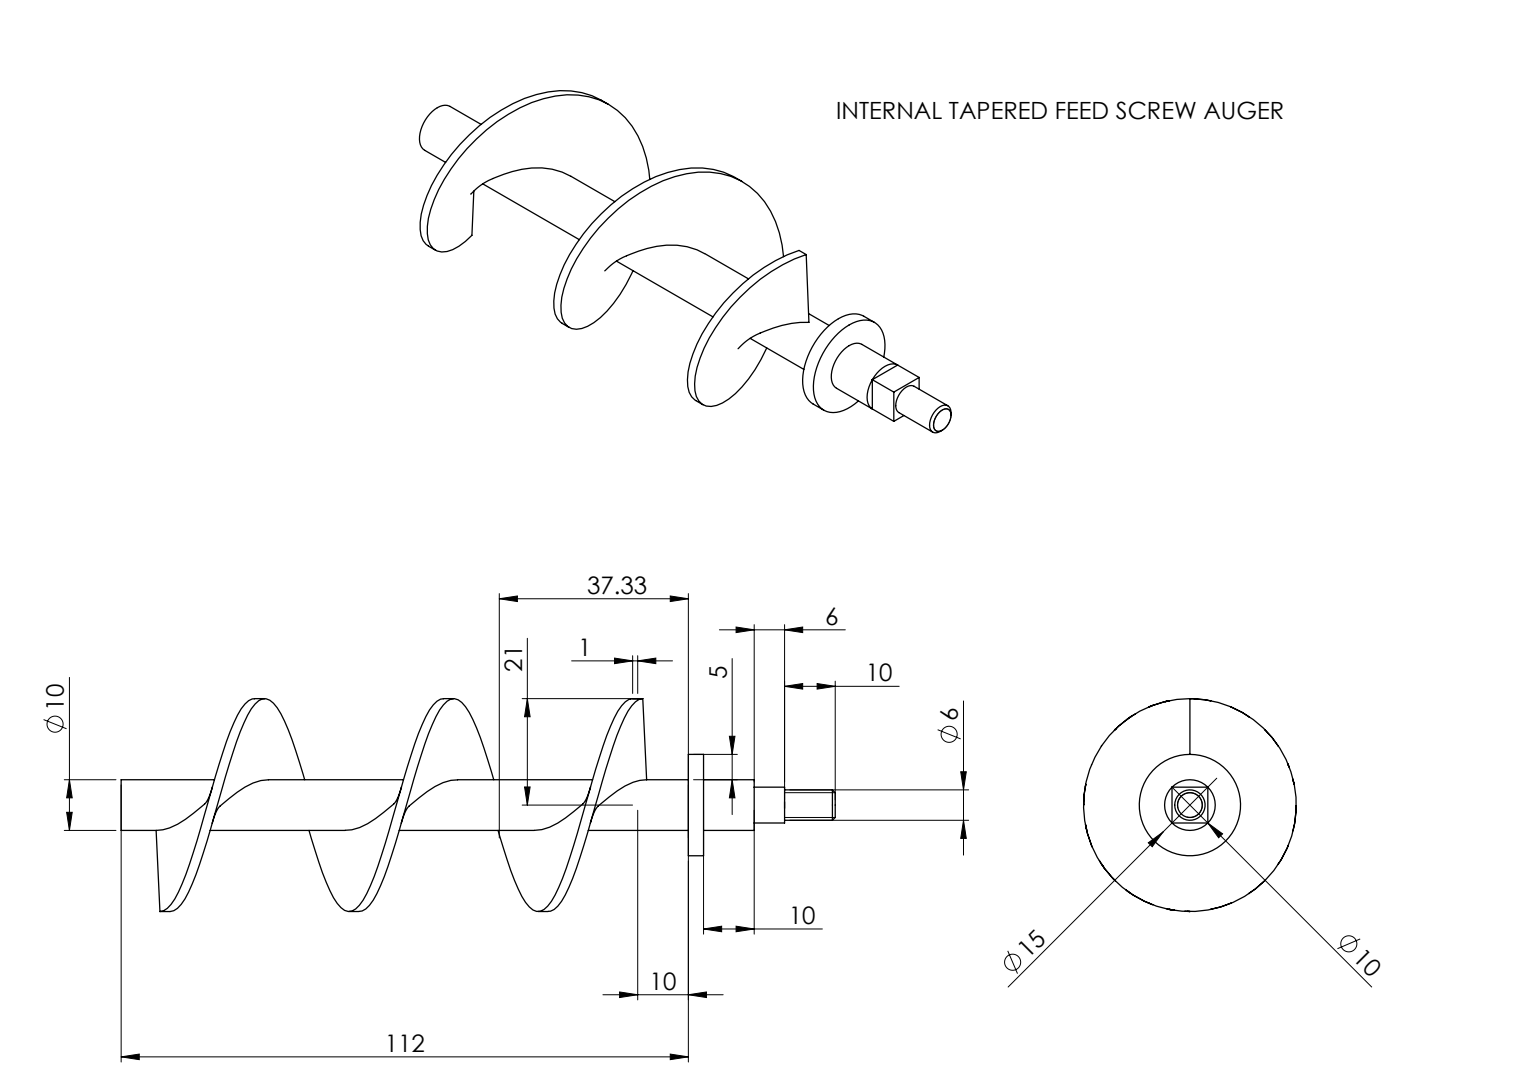
ISO-10303-21;
HEADER;
FILE_DESCRIPTION (('STEP AP214'),
    '1' );
FILE_NAME ('Internal Tapered Feed Screw Auger.step',
    '2026-10-22T10:02:39',
    ( '' ),
    ( '' ),
    'SwSTEP 2.0',
    'SolidWorks 2026',
    '' );
FILE_SCHEMA (( 'AUTOMOTIVE_DESIGN' ));
ENDSEC;

DATA;
#3=CARTESIAN_POINT ( 'NONE',  ( -24.57385867913225042, 55.01967498809302981, -0.01734603766092172178 ) ) ;
#8=CARTESIAN_POINT ( 'NONE',  ( -15.84874342590320673, 58.76832510134365606, 3.302529147201385129 ) ) ;
#12=CARTESIAN_POINT ( 'NONE',  ( 7.477680471578420196, 36.66673471410030061, 10.56605622896702990 ) ) ;
#17=CARTESIAN_POINT ( 'NONE',  ( 3.697305843545918513, 35.98616635274733255, -8.992456113074794644 ) ) ;
#18=EDGE_CURVE ( 'NONE', #2366, #7152, #6007, .T. ) ;
#22=CARTESIAN_POINT ( 'NONE',  ( 18.90732451447525975, 55.01449046109523522, 0.007799356525960917524 ) ) ;
#24=CARTESIAN_POINT ( 'NONE',  ( -46.47759630686348942, 71.80626330759284315, -12.92347896748408509 ) ) ;
#25=CARTESIAN_POINT ( 'NONE',  ( -13.52239577877046095, 75.98118489547775312, -2.745668029642679642 ) ) ;
#32=CARTESIAN_POINT ( 'NONE',  ( -54.99787500575298083, 55.00175321043320764, 0.0009066026748406779724 ) ) ;
#33=CARTESIAN_POINT ( 'NONE',  ( -34.13164850161200548, 51.02358645912743640, -3.048757558511538068 ) ) ;
#38=CARTESIAN_POINT ( 'NONE',  ( -1.477628194636992243, 49.49121550494065502, -20.47411891050684218 ) ) ;
#40=CARTESIAN_POINT ( 'NONE',  ( 10.96071222073927132, 53.39157304099641266, 4.745597011473480009 ) ) ;
#46=CARTESIAN_POINT ( 'NONE',  ( 3.204603673684104592, 51.02314964536983410, -3.048084100943247332 ) ) ;
#47=CARTESIAN_POINT ( 'NONE',  ( -28.33520174651890144, 42.04728119469179148, 5.364820852706460030 ) ) ;
#48=EDGE_CURVE ( 'NONE', #8851, #443, #4129, .T. ) ;
#59=CARTESIAN_POINT ( 'NONE',  ( -47.09272475956910142, 55.02483394329467359, -0.008490977716145282211 ) ) ;
#70=CARTESIAN_POINT ( 'NONE',  ( -62.96917444215183224, 46.00616310598284286, 19.01165851688606523 ) ) ;
#77=CARTESIAN_POINT ( 'NONE',  ( -27.49360061100878738, 37.45598436699922473, 11.71495266747331421 ) ) ;
#80=CARTESIAN_POINT ( 'NONE',  ( -12.37832547621337476, 59.49517489534859749, -2.213937092042313814 ) ) ;
#82=CARTESIAN_POINT ( 'NONE',  ( -3.477628190354089099, 49.49309465598528845, -20.46958112014059950 ) ) ;
#84=CARTESIAN_POINT ( 'NONE',  ( -23.14426256960421924, 52.25445662165124361, 21.02210202263520600 ) ) ;
#85=CARTESIAN_POINT ( 'NONE',  ( -68.81799204399976588, 34.52608862562686909, 5.501299279293338174 ) ) ;
#91=CARTESIAN_POINT ( 'NONE',  ( -44.20488284339200646, 55.00025175640378450, -0.002624240123811788852 ) ) ;
#92=CARTESIAN_POINT ( 'NONE',  ( -56.68145153021548310, 56.29769244905448744, 4.839614506206188160 ) ) ;
#94=CARTESIAN_POINT ( 'NONE',  ( 47.00000000000000000, 55.00000000000000000, 0.000000000000000000 ) ) ;
#95=CARTESIAN_POINT ( 'NONE',  ( -6.249156589778054105, 55.68730665650835476, -7.012895309292545676 ) ) ;
#108=CARTESIAN_POINT ( 'NONE',  ( -34.53957387867419015, 43.82314937793580611, -8.587433708483555250 ) ) ;
#121=CARTESIAN_POINT ( 'NONE',  ( -53.33538954556567546, 54.99810722428492937, -0.002143453996954131253 ) ) ;
#132=CARTESIAN_POINT ( 'NONE',  ( -6.160267096003628318, 59.12214581854949103, -20.69010011304746044 ) ) ;
#136=CARTESIAN_POINT ( 'NONE',  ( -6.214759040711413718, 65.81103152010582846, -18.03762937187994453 ) ) ;
#137=CARTESIAN_POINT ( 'NONE',  ( -46.52239103091250172, 73.32882989972571863, -10.56393531560676102 ) ) ;
#141=CARTESIAN_POINT ( 'NONE',  ( 46.99999999999999289, 58.53553390593273065, 3.535533905932731091 ) ) ;
#142=CARTESIAN_POINT ( 'NONE',  ( 4.636023424558444184, 34.00634798409771520, 1.031279783234476222 ) ) ;
#143=VECTOR ( 'NONE', #3904, 1000.000000000000000 ) ;
#145=CARTESIAN_POINT ( 'NONE',  ( -34.81092923608149192, 36.62878417468885317, -10.58136149031614970 ) ) ;
#146=CARTESIAN_POINT ( 'NONE',  ( -70.34104699118840642, 33.99562393659799397, 0.006612473344882377653 ) ) ;
#149=EDGE_CURVE ( 'NONE', #1776, #658, #10646, .T. ) ;
#151=EDGE_CURVE ( 'NONE', #658, #760, #3805, .T. ) ;
#154=CARTESIAN_POINT ( 'NONE',  ( -35.76380172564871884, 55.01086174631173975, 0.005834152228799136322 ) ) ;
#155=CARTESIAN_POINT ( 'NONE',  ( -44.62221111874860213, 58.76649436596603948, -3.304682393689729381 ) ) ;
#158=CARTESIAN_POINT ( 'NONE',  ( -6.833556764572190190, 56.37289815856257746, -6.894355924324841567 ) ) ;
#161=CARTESIAN_POINT ( 'NONE',  ( 9.477680475861957277, 36.67126955513442255, 10.56417786655960356 ) ) ;
#173=CARTESIAN_POINT ( 'NONE',  ( -30.96365390035560239, 40.99197526476194042, -0.6880654886566857087 ) ) ;
#181=EDGE_LOOP ( 'NONE', ( #6646, #3991, #9037, #3173 ) ) ;
#186=CARTESIAN_POINT ( 'NONE',  ( 6.125158419864718873, 48.06305152834397632, -1.028633690847041704 ) ) ;
#188=DIRECTION ( 'NONE',  ( 0.000000000000000000, 0.000000000000000000, 1.000000000000000000 ) ) ;
#194=CARTESIAN_POINT ( 'NONE',  ( -66.50782127702024127, 36.67013743889115318, 10.55179617378401247 ) ) ;
#197=EDGE_CURVE ( 'NONE', #1911, #3047, #4966, .T. ) ;
#199=CARTESIAN_POINT ( 'NONE',  ( -42.66281101964754896, 63.04450918361814615, -19.42252581123130639 ) ) ;
#200=AXIS2_PLACEMENT_3D ( 'NONE', #7923, #603, #5167 ) ;
#203=CARTESIAN_POINT ( 'NONE',  ( -30.99614452189004155, 33.97742542711323921, 0.0005215828242728561687 ) ) ;
#207=DIRECTION ( 'NONE',  ( -1.000000000000000000, -0.000000000000000000, -0.000000000000000000 ) ) ;
#210=CARTESIAN_POINT ( 'NONE',  ( -56.17294560383920299, 66.73154858138525469, 17.54339796666672058 ) ) ;
#212=CARTESIAN_POINT ( 'NONE',  ( -61.00490302436042356, 55.00059028654953153, 21.02810969917934614 ) ) ;
#215=VECTOR ( 'NONE', #1197, 1000.000000000000000 ) ;
#216=CARTESIAN_POINT ( 'NONE',  ( 53.00000000000000000, 51.46446609406726935, -3.535533905932738197 ) ) ;
#220=CARTESIAN_POINT ( 'NONE',  ( -14.57393009465980604, 54.98364064865898371, -0.001646604999752838971 ) ) ;
#224=CARTESIAN_POINT ( 'NONE',  ( 0.1668379413723253268, 49.14794564670181387, -3.906842406148068214 ) ) ;
#226=CARTESIAN_POINT ( 'NONE',  ( 14.14423903981857755, 49.50929293985068114, 20.43023407247793699 ) ) ;
#228=PLANE ( 'NONE',  #2565 ) ;
#237=CARTESIAN_POINT ( 'NONE',  ( -55.16972311799333539, 62.82217562642412645, 11.69677751401117405 ) ) ;
#246=CARTESIAN_POINT ( 'NONE',  ( -18.95794697780666027, 57.36371471763808927, 6.606639808170175598 ) ) ;
#251=CARTESIAN_POINT ( 'NONE',  ( 52.99999999999999289, 58.53553390593273065, 3.535533905932731091 ) ) ;
#253=CARTESIAN_POINT ( 'NONE',  ( -59.27472368810988002, 61.13901599248961105, 20.20251803659174783 ) ) ;
#256=CARTESIAN_POINT ( 'NONE',  ( -50.82691677660828589, 75.68920158268997511, 4.121780573430135597 ) ) ;
#262=PLANE ( 'NONE',  #3428 ) ;
#266=ADVANCED_FACE ( 'NONE', ( #3949 ), #228, .F. ) ;
#267=CARTESIAN_POINT ( 'NONE',  ( -58.49417186384191325, 59.10997037288393585, 20.69225924102262226 ) ) ;
#268=CARTESIAN_POINT ( 'NONE',  ( 14.87282114002693234, 58.67269055319452065, 13.65170787854068024 ) ) ;
#274=ORIENTED_EDGE ( 'NONE', *, *, #7349, .T. ) ;
#276=CARTESIAN_POINT ( 'NONE',  ( -68.24753854205350478, 55.02494518472502705, -0.0008082322394851507684 ) ) ;
#280=CARTESIAN_POINT ( 'NONE',  ( -69.87738456456679614, 41.01771127808763140, 1.829669757797043994 ) ) ;
#283=CARTESIAN_POINT ( 'NONE',  ( 36.99999999999999289, 59.99999999999998579, 0.000000000000000000 ) ) ;
#284=CARTESIAN_POINT ( 'NONE',  ( 53.00000000000000000, 51.46446609406726935, -3.535533905932738197 ) ) ;
#290=ORIENTED_EDGE ( 'NONE', *, *, #8254, .T. ) ;
#291=EDGE_CURVE ( 'NONE', #2366, #8948, #1373, .T. ) ;
#295=CARTESIAN_POINT ( 'NONE',  ( -53.99820501230367142, 64.90985867132549458, 9.909159326440711624 ) ) ;
#308=CARTESIAN_POINT ( 'NONE',  ( -24.89001229408545512, 50.71618230245203307, 5.579812370254800591 ) ) ;
#310=VECTOR ( 'NONE', #7758, 1000.000000000000227 ) ;
#316=CARTESIAN_POINT ( 'NONE',  ( -63.32723919479404628, 46.95276866351182576, 19.42062151208882170 ) ) ;
#319=CARTESIAN_POINT ( 'NONE',  ( -56.05785376386896246, 64.93131079446247611, 18.59685268580366468 ) ) ;
#321=CARTESIAN_POINT ( 'NONE',  ( -68.34104732181945963, 33.99448141944315438, 0.006743540747239065887 ) ) ;
#324=DIRECTION ( 'NONE',  ( 9.813077866773612233E-16, -1.000000000000000000, 0.000000000000000000 ) ) ;
#325=CARTESIAN_POINT ( 'NONE',  ( 15.18896243380506306, 60.50666922109576262, 20.46968130491651650 ) ) ;
#327=CARTESIAN_POINT ( 'NONE',  ( -61.99390593487224521, 46.95297697149054272, 19.42004845484624909 ) ) ;
#329=CARTESIAN_POINT ( 'NONE',  ( -61.59556246352555320, 52.94114603458827872, 20.93095456750423722 ) ) ;
#336=CARTESIAN_POINT ( 'NONE',  ( -70.57370072173033293, 55.01541170666005343, -0.006042036165150080004 ) ) ;
#339=DIRECTION ( 'NONE',  ( 0.000000000000000000, 0.000000000000000000, 1.000000000000000000 ) ) ;
#340=CARTESIAN_POINT ( 'NONE',  ( 2.791825101730443404, 48.06463389261614338, -1.028630067443766283 ) ) ;
#342=CARTESIAN_POINT ( 'NONE',  ( -28.67054321954914542, 35.57240153874681710, 8.046710727719679213 ) ) ;
#349=EDGE_CURVE ( 'NONE', #1114, #2366, #8625, .T. ) ;
#353=CARTESIAN_POINT ( 'NONE',  ( -58.37019661190561948, 55.68797971655733647, 13.99244826128962593 ) ) ;
#365=EDGE_CURVE ( 'NONE', #1817, #1911, #2263, .T. ) ;
#366=CARTESIAN_POINT ( 'NONE',  ( 5.249530852090826372, 48.30269735457433455, -2.031231156380094660 ) ) ;
#374=ADVANCED_FACE ( 'NONE', ( #6893 ), #4791, .T. ) ;
#376=CARTESIAN_POINT ( 'NONE',  ( -59.82750509709391196, 59.10995506582904824, 20.69284243654335498 ) ) ;
#380=CARTESIAN_POINT ( 'NONE',  ( -59.59556320886013481, 52.94111634316250559, 20.93276532467568174 ) ) ;
#387=CARTESIAN_POINT ( 'NONE',  ( -9.070746587277097817, 68.33487957594263662, -16.24597445391072270 ) ) ;
#389=CARTESIAN_POINT ( 'NONE',  ( 18.18897147127288605, 67.92208482572254979, 16.80535131051722075 ) ) ;
#390=CARTESIAN_POINT ( 'NONE',  ( -3.793771210778672298, 51.32715215846550905, -13.65164055122976983 ) ) ;
#391=DIRECTION ( 'NONE',  ( 6.033820786006286457E-17, -1.000000000000000000, 0.000000000000000000 ) ) ;
#403=CARTESIAN_POINT ( 'NONE',  ( -32.20817489827727087, 48.19891751814265035, 1.703719440855944844 ) ) ;
#405=CARTESIAN_POINT ( 'NONE',  ( -27.49360061100878738, 37.45598436699922473, 11.71495266747331421 ) ) ;
#414=ORIENTED_EDGE ( 'NONE', *, *, #3400, .F. ) ;
#415=CARTESIAN_POINT ( 'NONE',  ( -23.18906244097991021, 49.50939288222085821, 20.43027456479002879 ) ) ;
#428=CARTESIAN_POINT ( 'NONE',  ( -8.750920173525754464, 61.18660372065389907, -3.306409054201195907 ) ) ;
#434=ORIENTED_EDGE ( 'NONE', *, *, #8927, .T. ) ;
#435=CARTESIAN_POINT ( 'NONE',  ( -42.92935705524211443, 57.05913440163546113, -20.93112575922673102 ) ) ;
#443=VERTEX_POINT ( 'NONE', #7009 ) ;
#446=CARTESIAN_POINT ( 'NONE',  ( -32.99614454614441428, 33.97685596767119165, 0.0005149883856687357403 ) ) ;
#449=CARTESIAN_POINT ( 'NONE',  ( -60.26222962708032327, 52.94112624030389469, 20.93216173895077503 ) ) ;
#450=CARTESIAN_POINT ( 'NONE',  ( -25.53957388397973105, 51.34093700237838931, 13.61837799178155350 ) ) ;
#457=CARTESIAN_POINT ( 'NONE',  ( -64.61922394917361601, 54.99794615529658159, 0.004759334053694205813 ) ) ;
#458=VECTOR ( 'NONE', #2991, 1000.000000000000000 ) ;
#461=CARTESIAN_POINT ( 'NONE',  ( -22.00013559226026771, 57.68156399829890546, 6.473040822733857169 ) ) ;
#462=ORIENTED_EDGE ( 'NONE', *, *, #11425, .T. ) ;
#463=CARTESIAN_POINT ( 'NONE',  ( -30.40408068685511367, 34.08504365610654219, 2.058398070974400529 ) ) ;
#473=CARTESIAN_POINT ( 'NONE',  ( -7.070747353360942178, 68.33360022464046324, -16.24461469319379603 ) ) ;
#482=DIRECTION ( 'NONE',  ( -9.813077866773612233E-16, 1.000000000000000000, 0.000000000000000000 ) ) ;
#486=CARTESIAN_POINT ( 'NONE',  ( -60.95809730739352261, 51.99959260526208737, 6.342595581606403243 ) ) ;
#496=LINE ( 'NONE', #7937, #10551 ) ;
#497=CARTESIAN_POINT ( 'NONE',  ( 10.42614132098574586, 55.02481535990867911, -0.008496357143309388182 ) ) ;
#501=CARTESIAN_POINT ( 'NONE',  ( -41.16026710375170694, 50.89060761561553647, -20.69263693287480521 ) ) ;
#503=CARTESIAN_POINT ( 'NONE',  ( -68.19377681732581209, 34.02207046653818168, 2.749122354329981643 ) ) ;
#504=CARTESIAN_POINT ( 'NONE',  ( -41.49691193415848289, 52.26032216745779380, -13.79378832249819986 ) ) ;
#507=CARTESIAN_POINT ( 'NONE',  ( -27.14812531749841895, 52.78402274155275364, 4.494092492992627363 ) ) ;
#511=CARTESIAN_POINT ( 'NONE',  ( -69.75702627179666138, 54.98186149566993208, 0.007223337549123830421 ) ) ;
#514=CIRCLE ( 'NONE', #703, 2.999999999999995559 ) ;
#516=CARTESIAN_POINT ( 'NONE',  ( -50.77658096445664171, 61.83369931620287474, -1.838789935413423171 ) ) ;
#519=CARTESIAN_POINT ( 'NONE',  ( -54.32961274566940801, 69.86573439484330095, 14.86481071665870601 ) ) ;
#531=CARTESIAN_POINT ( 'NONE',  ( -5.030643890195627854, 62.08057558410310861, -19.78873666113293694 ) ) ;
#536=ORIENTED_EDGE ( 'NONE', *, *, #5953, .F. ) ;
#539=DIRECTION ( 'NONE',  ( -1.000000000000000000, -6.033820786006286457E-17, -0.000000000000000000 ) ) ;
#543=CARTESIAN_POINT ( 'NONE',  ( -53.95794482029891981, 59.71207155077219397, 5.199202863523991525 ) ) ;
#553=CARTESIAN_POINT ( 'NONE',  ( -18.33546440020741741, 54.99907998473290149, -0.002823738427829867569 ) ) ;
#561=CARTESIAN_POINT ( 'NONE',  ( -40.60828084101493829, 48.86090744392433294, -20.20262880343927847 ) ) ;
#563=CARTESIAN_POINT ( 'NONE',  ( -60.92889604530372338, 52.94113613744689673, 20.93155815322914393 ) ) ;
#564=CARTESIAN_POINT ( 'NONE',  ( -11.16981900506391234, 66.69595144640879880, -7.821387473301188997 ) ) ;
#567=VERTEX_POINT ( 'NONE', #5147 ) ;
#569=CARTESIAN_POINT ( 'NONE',  ( 16.47760469315713294, 57.74566955740679930, 20.97627666568605420 ) ) ;
#573=CARTESIAN_POINT ( 'NONE',  ( 19.14254474247333349, 57.21240123512449571, 4.495849551821894607 ) ) ;
#574=CARTESIAN_POINT ( 'NONE',  ( -25.10988330751693809, 54.08371348254146938, 7.017189493341159157 ) ) ;
#576=CARTESIAN_POINT ( 'NONE',  ( -36.47762819585614835, 42.07544065584382764, -16.80749884933775462 ) ) ;
#588=CARTESIAN_POINT ( 'NONE',  ( -18.73741402030934111, 64.90551912913463184, 18.53518525054827393 ) ) ;
#593=CARTESIAN_POINT ( 'NONE',  ( 36.99999999999999289, 55.00000000000000000, 0.000000000000000000 ) ) ;
#603=DIRECTION ( 'NONE',  ( 1.000000000000000000, 0.000000000000000000, 0.000000000000000000 ) ) ;
#606=CARTESIAN_POINT ( 'NONE',  ( -49.58248963817779753, 62.01904108894438394, 0.6873064985993181386 ) ) ;
#607=CARTESIAN_POINT ( 'NONE',  ( 47.00000000000000000, 55.00000000000000000, 0.000000000000000000 ) ) ;
#616=FACE_BOUND ( 'NONE', #1270, .T. ) ;
#617=CARTESIAN_POINT ( 'NONE',  ( 25.99999999999999645, 54.99999999999999289, 0.000000000000000000 ) ) ;
#620=CARTESIAN_POINT ( 'NONE',  ( -29.45688395272410887, 50.03307866788530589, 0.6599468027641450796 ) ) ;
#621=CARTESIAN_POINT ( 'NONE',  ( -42.03064326886630653, 53.96872019721284630, -20.99365203016559178 ) ) ;
#623=CARTESIAN_POINT ( 'NONE',  ( -45.17314290467847115, 66.71834769317766245, -17.55197735385382174 ) ) ;
#624=CARTESIAN_POINT ( 'NONE',  ( -30.70300456119418797, 42.33444820903851991, 5.990538379293029791 ) ) ;
#634=CARTESIAN_POINT ( 'NONE',  ( -11.49982872529378852, 60.84893598204366327, -3.911509378443825291 ) ) ;
#636=CARTESIAN_POINT ( 'NONE',  ( -61.63584152524990145, 46.00569487729882212, 19.01260273971552905 ) ) ;
#637=CARTESIAN_POINT ( 'NONE',  ( 19.14436220527237253, 71.77763100192429135, 12.89423484158165500 ) ) ;
#639=ADVANCED_FACE ( 'NONE', ( #8250 ), #10934, .T. ) ;
#647=CARTESIAN_POINT ( 'NONE',  ( 14.85570562722353749, 52.25434861561973321, 21.02374011750137939 ) ) ;
#652=CARTESIAN_POINT ( 'NONE',  ( -32.11869219899978845, 34.20636958863568822, 3.085052597841025701 ) ) ;
#658=VERTEX_POINT ( 'NONE', #3636 ) ;
#659=CARTESIAN_POINT ( 'NONE',  ( -66.89547590671475064, 48.02433609231711387, 0.9101378528334346241 ) ) ;
#672=CARTESIAN_POINT ( 'NONE',  ( 22.90732450365403849, 55.02356608025330331, 0.01155963734724412169 ) ) ;
#677=CARTESIAN_POINT ( 'NONE',  ( -54.59603348275399526, 73.54984634329692028, 9.912388241271610667 ) ) ;
#678=VERTEX_POINT ( 'NONE', #4538 ) ;
#679=CARTESIAN_POINT ( 'NONE',  ( -23.81092923484322199, 52.25445676425606223, 21.02046492383515641 ) ) ;
#680=CARTESIAN_POINT ( 'NONE',  ( -44.99813998784102154, 60.36285607543581477, -12.94816624433304142 ) ) ;
#682=CIRCLE ( 'NONE', #1258, 2.445500000000003116 ) ;
#684=MANIFOLD_SOLID_BREP ( 'M6 Machine Threads Stud1', #2327 ) ;
#690=CARTESIAN_POINT ( 'NONE',  ( -70.99971551311861617, 47.99600105715470733, 0.0002324378226963109213 ) ) ;
#691=ORIENTED_EDGE ( 'NONE', *, *, #8944, .T. ) ;
#692=CARTESIAN_POINT ( 'NONE',  ( -61.32723930490969622, 46.95308112547827051, 19.41976192622660946 ) ) ;
#702=CARTESIAN_POINT ( 'NONE',  ( -54.63607242817042930, 69.12530316040908929, 15.58420556269393309 ) ) ;
#703=AXIS2_PLACEMENT_3D ( 'NONE', #8408, #9360, #5659 ) ;
#712=LINE ( 'NONE', #6193, #3438 ) ;
#717=CARTESIAN_POINT ( 'NONE',  ( -37.91582326205369213, 52.94892034820053084, -6.747764776534440401 ) ) ;
#729=CARTESIAN_POINT ( 'NONE',  ( 9.097072198540729460, 54.98136927407220753, 0.006368393940946715480 ) ) ;
#732=CARTESIAN_POINT ( 'NONE',  ( -10.79095582353838090, 59.95900821267746750, -0.6598374012892626039 ) ) ;
#737=CARTESIAN_POINT ( 'NONE',  ( -31.45202553487676411, 34.20668501241195969, 3.085052028771560373 ) ) ;
#743=CARTESIAN_POINT ( 'NONE',  ( 14.85570562722353749, 52.25434861561973321, 21.02374011750137939 ) ) ;
#746=CARTESIAN_POINT ( 'NONE',  ( 7.876834456762007441, 50.04083008229487461, 0.6585545532920904499 ) ) ;
#747=CARTESIAN_POINT ( 'NONE',  ( 11.09270675091795511, 55.00778140979137021, -0.01448337108733858611 ) ) ;
#750=CARTESIAN_POINT ( 'NONE',  ( 4.214641129381988094, 34.60917520197180153, -5.106920541952282733 ) ) ;
#751=CARTESIAN_POINT ( 'NONE',  ( -4.188986194789085182, 52.25407379690145859, -20.98118322582191908 ) ) ;
#759=CARTESIAN_POINT ( 'NONE',  ( -64.47562408583945626, 38.19583575827792288, 12.92744520505189953 ) ) ;
#760=VERTEX_POINT ( 'NONE', #10090 ) ;
#764=ORIENTED_EDGE ( 'NONE', *, *, #8944, .F. ) ;
#767=CARTESIAN_POINT ( 'NONE',  ( -67.17448730496187181, 36.66801277209461318, 10.55271442276269944 ) ) ;
#774=CARTESIAN_POINT ( 'NONE',  ( -2.626967639481237349, 55.33059824256177706, -5.000002997081709921 ) ) ;
#775=CARTESIAN_POINT ( 'NONE',  ( 21.46051530992876977, 66.17699122582456539, 8.587284035366270274 ) ) ;
#788=CARTESIAN_POINT ( 'NONE',  ( -43.43046782438146636, 54.98524932194441561, 0.01300693185584521350 ) ) ;
#792=CARTESIAN_POINT ( 'NONE',  ( -21.29436769408802377, 54.66877947394643655, 4.999995929924349269 ) ) ;
#793=CARTESIAN_POINT ( 'NONE',  ( -68.81799204399976588, 34.52608862562686909, 5.501299279293338174 ) ) ;
#795=CARTESIAN_POINT ( 'NONE',  ( -43.11869212536358020, 60.10704077131471479, -20.39111636944713624 ) ) ;
#802=CARTESIAN_POINT ( 'NONE',  ( 0.8557374297261139962, 42.07536394375442512, -16.80742094040031631 ) ) ;
#806=CARTESIAN_POINT ( 'NONE',  ( -9.204882831600160742, 55.00123686646767851, -0.002328140736296190928 ) ) ;
#808=ADVANCED_FACE ( 'NONE', ( #9564 ), #5862, .T. ) ;
#809=CARTESIAN_POINT ( 'NONE',  ( 11.85573742417284748, 44.41863851231033067, 18.37121583117139778 ) ) ;
#810=CARTESIAN_POINT ( 'NONE',  ( -7.929357056070021947, 64.91238717040420170, -18.54984206437098493 ) ) ;
#819=DIRECTION ( 'NONE',  ( 1.000000000000000000, 6.033820786006286457E-17, -0.000000000000000000 ) ) ;
#820=CARTESIAN_POINT ( 'NONE',  ( -60.98114229612854587, 55.65873833719333419, 4.967062080433862548 ) ) ;
#830=CARTESIAN_POINT ( 'NONE',  ( -6.455306493259947764, 63.34608869971732048, -11.25480877436020855 ) ) ;
#835=B_SPLINE_CURVE_WITH_KNOTS ( 'NONE', 3,
 ( #2892, #1982, #4749, #2043, #8400, #3851, #7516, #2952, #9062, #6740, #4029, #2165, #11199, #9414, #8645, #2105, #7686, #5895, #6859, #7628, #3970, #11321, #8701, #5053, #5835, #9536, #3245, #11259, #9475, #1263, #4141, #4085, #3070, #4932, #7803, #5778, #6796, #1392 ),
 .UNSPECIFIED., .F., .F.,
 ( 4, 2, 2, 2, 2, 2, 2, 2, 2, 2, 2, 2, 2, 2, 2, 2, 2, 2, 4 ),
 ( 0.07285479446859771668, 0.07361368492618262926, 0.07437257538376754185, 0.07589035629893736701, 0.07740813721410717829, 0.07892591812927700345, 0.08044369904444681474, 0.08196147995961662602, 0.08347926087478645119, 0.08499704178995626247, 0.08575593224754117505, 0.08651482270512608763, 0.08803260362029592667, 0.08955038453546575183, 0.09106816545063559087, 0.09258594636580541604, 0.09410372728097524120, 0.09562150819614508024, 0.09713928911131490540 ),
 .UNSPECIFIED. ) ;
#842=CARTESIAN_POINT ( 'NONE',  ( -38.17020195889585921, 54.99973427304116314, 0.005832240597639265153 ) ) ;
#846=CARTESIAN_POINT ( 'NONE',  ( -20.12390779004163477, 55.65879866787057750, 4.959133026351390860 ) ) ;
#848=CARTESIAN_POINT ( 'NONE',  ( -63.32723919479404628, 46.95276866351182576, 19.42062151208882170 ) ) ;
#850=CARTESIAN_POINT ( 'NONE',  ( -13.52239577877046095, 75.98118489547775312, -2.745668029642679642 ) ) ;
#856=CARTESIAN_POINT ( 'NONE',  ( -29.26269115883859939, 34.87241548204915631, 6.108265559058850158 ) ) ;
#860=CARTESIAN_POINT ( 'NONE',  ( -60.50017553191300834, 56.37004246370271687, 6.895233585243415675 ) ) ;
#863=CARTESIAN_POINT ( 'NONE',  ( 20.47769554116023372, 71.77531707407277395, 12.89192088424961824 ) ) ;
#864=CARTESIAN_POINT ( 'NONE',  ( -8.785358865379802040, 67.52185545713140868, -16.88477868139494831 ) ) ;
#869=EDGE_CURVE ( 'NONE', #8948, #11420, #9501, .T. ) ;
#871=CARTESIAN_POINT ( 'NONE',  ( 47.00000000000000000, 55.00000000000000000, 0.000000000000000000 ) ) ;
#872=CARTESIAN_POINT ( 'NONE',  ( -13.75936034494452542, 55.01575878706701417, -0.004732648836832428763 ) ) ;
#873=CARTESIAN_POINT ( 'NONE',  ( -55.12858368788357666, 57.50315721827126936, 4.331434029952367482 ) ) ;
#875=CARTESIAN_POINT ( 'NONE',  ( 34.00000000000000000, 55.00000000000000000, 0.000000000000000000 ) ) ;
#876=AXIS2_PLACEMENT_3D ( 'NONE', #2832, #11141, #188 ) ;
#882=CARTESIAN_POINT ( 'NONE',  ( 19.12485590497331245, 59.33891611993333726, 2.506220315686558564 ) ) ;
#890=CARTESIAN_POINT ( 'NONE',  ( -3.262052055525263228, 56.37336850891590956, -14.01842231928934090 ) ) ;
#899=EDGE_CURVE ( 'NONE', #3592, #7749, #2919, .T. ) ;
#901=CARTESIAN_POINT ( 'NONE',  ( -31.76380171923032947, 55.01766230220479059, 0.008650971149387511397 ) ) ;
#909=CARTESIAN_POINT ( 'NONE',  ( -15.14429485721040614, 76.01882847486140804, 2.745652427074330326 ) ) ;
#915=CARTESIAN_POINT ( 'NONE',  ( 2.274842917244503937, 38.70728229458904934, -13.38060881307704975 ) ) ;
#921=CARTESIAN_POINT ( 'NONE',  ( -64.29142959965328430, 52.00076317697213568, 6.340235024524601748 ) ) ;
#923=CARTESIAN_POINT ( 'NONE',  ( -41.59602423483332956, 57.05917253807995593, -20.93237218927098198 ) ) ;
#925=CARTESIAN_POINT ( 'NONE',  ( -7.337209909475700620, 63.04728967918421745, -19.42673836724018699 ) ) ;
#927=DIRECTION ( 'NONE',  ( 6.033820786006286457E-17, -1.000000000000000000, 0.000000000000000000 ) ) ;
#934=CARTESIAN_POINT ( 'NONE',  ( -31.66451884688278184, 54.99809435283415837, 0.0005903141131624571472 ) ) ;
#935=CARTESIAN_POINT ( 'NONE',  ( -53.18446182085578045, 58.76752042146932098, 3.303451655433074396 ) ) ;
#941=CARTESIAN_POINT ( 'NONE',  ( -9.391823749396904120, 73.59702374900430755, -9.931971109272440756 ) ) ;
#943=CARTESIAN_POINT ( 'NONE',  ( 17.18511958428734232, 58.30390285059421984, 3.767129572935171034 ) ) ;
#951=CARTESIAN_POINT ( 'NONE',  ( -5.349432795815419084, 57.50648965827332404, -4.338654380549343159 ) ) ;
#952=CARTESIAN_POINT ( 'NONE',  ( -28.03633875861160263, 42.33641998042576660, 5.989639417439852842 ) ) ;
#966=CARTESIAN_POINT ( 'NONE',  ( -44.75936011935566228, 55.01969457619907899, -0.01734821724329012674 ) ) ;
#970=CARTESIAN_POINT ( 'NONE',  ( -20.71005862496660654, 55.16551809362240988, 5.000002034471375367 ) ) ;
#975=CARTESIAN_POINT ( 'NONE',  ( 10.52240409369262153, 44.41989175727180594, 18.36819097564579195 ) ) ;
#982=CARTESIAN_POINT ( 'NONE',  ( -23.18906244097991021, 49.50939288222085821, 20.43027456479002879 ) ) ;
#984=CARTESIAN_POINT ( 'NONE',  ( -60.45014771802851072, 49.89223742090062075, 20.38901927491476584 ) ) ;
#986=CARTESIAN_POINT ( 'NONE',  ( -8.287358458837889685, 57.06376126929644954, -4.557158438297962633 ) ) ;
#987=CARTESIAN_POINT ( 'NONE',  ( -1.144262565995328940, 42.07883645215377300, -16.80394782698530065 ) ) ;
#989=CARTESIAN_POINT ( 'NONE',  ( -45.05849143660482525, 68.38147613270652414, -16.29358623752561641 ) ) ;
#990=CARTESIAN_POINT ( 'NONE',  ( -11.39182375260447166, 73.60042400440836730, -9.933379572949093017 ) ) ;
#997=CARTESIAN_POINT ( 'NONE',  ( 34.00000000000000000, 50.00000000000001421, 6.123233995736750505E-16 ) ) ;
#998=CARTESIAN_POINT ( 'NONE',  ( -44.79520175934491988, 54.99837535002616562, 0.003324556147400343012 ) ) ;
#999=CARTESIAN_POINT ( 'NONE',  ( -63.28902608371529936, 51.23315991719264417, 3.304235638531133112 ) ) ;
#1002=CARTESIAN_POINT ( 'NONE',  ( 20.77652457878251013, 61.80192317012852499, 1.825703622701588813 ) ) ;
#1004=CARTESIAN_POINT ( 'NONE',  ( 6.636022776496402820, 34.00797225689733239, 1.031222807066483504 ) ) ;
#1007=CARTESIAN_POINT ( 'NONE',  ( 5.126123443351389142, 50.15990383064929858, 1.295883551324225946 ) ) ;
#1013=CARTESIAN_POINT ( 'NONE',  ( -42.63032052581742448, 60.99632860981928673, -12.67841600781651046 ) ) ;
#1022=AXIS2_PLACEMENT_3D ( 'NONE', #7611, #11239, #3051 ) ;
#1025=CARTESIAN_POINT ( 'NONE',  ( -31.16317214572511674, 54.99555836494509720, -0.0001888778372106834306 ) ) ;
#1028=ORIENTED_EDGE ( 'NONE', *, *, #10581, .T. ) ;
#1034=CARTESIAN_POINT ( 'NONE',  ( -62.66057256483475868, 46.95287281750281494, 19.42033498346916787 ) ) ;
#1037=CARTESIAN_POINT ( 'NONE',  ( -16.69731055678936826, 70.57278980777935828, 14.11442052818484783 ) ) ;
#1038=( NAMED_UNIT ( * ) SI_UNIT ( $, .STERADIAN. ) SOLID_ANGLE_UNIT ( ) );
#1039=CARTESIAN_POINT ( 'NONE',  ( -43.83980969374544401, 66.71858909844225138, -17.55257377017560216 ) ) ;
#1042=CARTESIAN_POINT ( 'NONE',  ( 1.046276059170544448, 50.44260135563150271, -2.063240075633586024 ) ) ;
#1043=COLOUR_RGB ( '',0.8941176470588234615, 0.8941176470588234615, 0.8941176470588234615 ) ;
#1044=CARTESIAN_POINT ( 'NONE',  ( 14.47760468889531182, 57.74566952947367326, 20.98118467575540436 ) ) ;
#1047=CARTESIAN_POINT ( 'NONE',  ( -42.45202546124224341, 60.10692058874730037, -20.39082473449001043 ) ) ;
#1048=CARTESIAN_POINT ( 'NONE',  ( -50.14429338685609849, 75.46958046783008456, -5.506903914760000518 ) ) ;
#1056=CARTESIAN_POINT ( 'NONE',  ( -16.90719202101858087, 54.98551469821890691, -0.007782449515281230322 ) ) ;
#1057=CARTESIAN_POINT ( 'NONE',  ( -50.46075028443474508, 59.84060402248204014, 1.293943614083152394 ) ) ;
#1059=CARTESIAN_POINT ( 'NONE',  ( -56.07732272482616764, 65.82928010674932295, 8.888286616055713907 ) ) ;
#1071=CARTESIAN_POINT ( 'NONE',  ( -61.29696941632089846, 49.00264374128124700, 12.67759916065936743 ) ) ;
#1073=AXIS2_PLACEMENT_3D ( 'NONE', #1210, #2957, #3857 ) ;
#1078=ORIENTED_EDGE ( 'NONE', *, *, #7905, .F. ) ;
#1086=CARTESIAN_POINT ( 'NONE',  ( -5.249611880419077892, 58.30742012212186154, -6.189572715011546933 ) ) ;
#1090=ORIENTED_EDGE ( 'NONE', *, *, #6143, .T. ) ;
#1095=CARTESIAN_POINT ( 'NONE',  ( 23.00000000000000000, 76.00000000000000000, 0.000000000000000000 ) ) ;
#1099=CARTESIAN_POINT ( 'NONE',  ( -54.32961274566940801, 69.86573439484330095, 14.86481071665870601 ) ) ;
#1100=CARTESIAN_POINT ( 'NONE',  ( -50.82691677660828589, 75.68920158268997511, 4.121780573430135597 ) ) ;
#1103=DIRECTION ( 'NONE',  ( 0.000000000000000000, 0.000000000000000000, 1.000000000000000000 ) ) ;
#1106=CARTESIAN_POINT ( 'NONE',  ( -18.26269090243636128, 68.34536746166378407, 16.25747718207173520 ) ) ;
#1107=CARTESIAN_POINT ( 'NONE',  ( 7.127167418523728593, 42.78307170200208276, 7.042457608538825298 ) ) ;
#1114=VERTEX_POINT ( 'NONE', #1204 ) ;
#1116=CARTESIAN_POINT ( 'NONE',  ( -25.42602701123318099, 54.99834177037958938, 0.01637032750073019391 ) ) ;
#1117=CARTESIAN_POINT ( 'NONE',  ( -36.46296276145401549, 52.49655656964354478, -4.331271186457903433 ) ) ;
#1119=CARTESIAN_POINT ( 'NONE',  ( -69.13100345326250817, 41.34467958230499107, 3.669940632046716278 ) ) ;
#1122=CARTESIAN_POINT ( 'NONE',  ( -5.929357825456832209, 64.91315550346766372, -18.55154749960842153 ) ) ;
#1133=CARTESIAN_POINT ( 'NONE',  ( -36.12710455038816093, 46.37784419364835742, -11.21156427467630223 ) ) ;
#1144=CARTESIAN_POINT ( 'NONE',  ( 0.7765813511237322775, 51.48435031992290334, -6.093068385610369120 ) ) ;
#1154=CARTESIAN_POINT ( 'NONE',  ( -42.33720994522852266, 55.00043528610386545, -21.02753041772728437 ) ) ;
#1164=CARTESIAN_POINT ( 'NONE',  ( -8.481641943402102868, 57.21203007224725212, -4.487076300782732119 ) ) ;
#1166=CARTESIAN_POINT ( 'NONE',  ( 3.451907635234679361, 34.19915017745972108, -3.085386652995293133 ) ) ;
#1169=CARTESIAN_POINT ( 'NONE',  ( -53.54812715265580181, 73.03736663818040142, 10.81090271242882039 ) ) ;
#1170=AXIS2_PLACEMENT_3D ( 'NONE', #593, #1385, #5046 ) ;
#1171=CARTESIAN_POINT ( 'NONE',  ( 21.12703399079512323, 68.61832863460267617, 3.659187381993185717 ) ) ;
#1179=CARTESIAN_POINT ( 'NONE',  ( -63.46281172795519154, 55.00260107563563139, -0.003976208690220505923 ) ) ;
#1186=CARTESIAN_POINT ( 'NONE',  ( -55.78867880362859921, 66.25575517429669503, 8.346979382912829593 ) ) ;
#1187=EDGE_LOOP ( 'NONE', ( #9606, #9183 ) ) ;
#1188=CARTESIAN_POINT ( 'NONE',  ( -4.160267277967630406, 59.12176995062825569, -20.68921489609442332 ) ) ;
#1195=VERTEX_POINT ( 'NONE', #7671 ) ;
#1197=DIRECTION ( 'NONE',  ( -1.000000000000000000, -6.033820786006286457E-17, -0.000000000000000000 ) ) ;
#1199=CARTESIAN_POINT ( 'NONE',  ( -67.21123314643752167, 41.02399581862376721, 1.828645404196747037 ) ) ;
#1204=CARTESIAN_POINT ( 'NONE',  ( 52.99999999999999289, 58.53553390593273065, -3.535533905932738197 ) ) ;
#1207=ORIENTED_EDGE ( 'NONE', *, *, #3224, .T. ) ;
#1208=CARTESIAN_POINT ( 'NONE',  ( -16.04203362689861834, 60.18690525748159814, 4.700552706782350931 ) ) ;
#1210=CARTESIAN_POINT ( 'NONE',  ( 52.99999999999999289, 55.00000000000000000, 0.000000000000000000 ) ) ;
#1215=CARTESIAN_POINT ( 'NONE',  ( -53.69727390230763575, 74.79022971164903311, 7.081167078663678893 ) ) ;
#1218=CARTESIAN_POINT ( 'NONE',  ( -54.63607242817042930, 69.12530316040908929, 15.58420556269393309 ) ) ;
#1222=CARTESIAN_POINT ( 'NONE',  ( -6.544209565228709558, 55.65803961495722518, -4.967200339763780725 ) ) ;
#1224=ORIENTED_EDGE ( 'NONE', *, *, #197, .F. ) ;
#1226=CARTESIAN_POINT ( 'NONE',  ( -61.40197252463548239, 48.89621197884387982, 20.10936848441244607 ) ) ;
#1227=CARTESIAN_POINT ( 'NONE',  ( 9.460426116349054837, 46.40793895553105131, 11.18147790519370766 ) ) ;
#1230=CARTESIAN_POINT ( 'NONE',  ( -18.99070286106124428, 58.97347284273117651, 3.052796309671656161 ) ) ;
#1238=CARTESIAN_POINT ( 'NONE',  ( 1.042054107055792711, 48.65947148651063259, -2.999074899036769271 ) ) ;
#1240=CARTESIAN_POINT ( 'NONE',  ( -15.82693394478133797, 72.53700911420227726, 11.72543866452437733 ) ) ;
#1248=ORIENTED_EDGE ( 'NONE', *, *, #10185, .F. ) ;
#1252=CARTESIAN_POINT ( 'NONE',  ( -36.87283257201146114, 47.96004688000734006, -12.21088183946608119 ) ) ;
#1258=AXIS2_PLACEMENT_3D ( 'NONE', #7063, #7123, #10746 ) ;
#1263=CARTESIAN_POINT ( 'NONE',  ( -48.15199486393218109, 58.76922744225378636, -3.301526873569539777 ) ) ;
#1266=CARTESIAN_POINT ( 'NONE',  ( -4.666526940154917646, 57.68340530217055573, -6.477642677762205814 ) ) ;
#1270=EDGE_LOOP ( 'NONE', ( #9513, #11457 ) ) ;
#1275=CARTESIAN_POINT ( 'NONE',  ( -60.69833702282029009, 56.03208645306531110, 20.99415308669729541 ) ) ;
#1286=CARTESIAN_POINT ( 'NONE',  ( -45.83980951013849392, 66.71822699054862937, -17.55167914569291554 ) ) ;
#1288=CARTESIAN_POINT ( 'NONE',  ( -1.189062444204875835, 44.43480771519530492, -18.33185415547853481 ) ) ;
#1289=VECTOR ( 'NONE', #8219, 1000.000000000000000 ) ;
#1290=CARTESIAN_POINT ( 'NONE',  ( -43.21475900837984341, 58.08538667521604282, -20.80084980650556759 ) ) ;
#1292=DIRECTION ( 'NONE',  ( 1.000000000000000000, 6.033820786006286457E-17, 0.000000000000000000 ) ) ;
#1298=DIRECTION ( 'NONE',  ( -0.04813578311308589625, -0.9988407004187033200, 0.0004489667737563936712 ) ) ;
#1302=CARTESIAN_POINT ( 'NONE',  ( -31.91627726477343074, 48.28752732786880841, 2.036885257361992441 ) ) ;
#1304=CARTESIAN_POINT ( 'NONE',  ( -53.73751484135783585, 71.24472392590685388, 13.33357819947211453 ) ) ;
#1315=CARTESIAN_POINT ( 'NONE',  ( -1.477628194636992243, 49.49121550494065502, -20.47411891050684218 ) ) ;
#1323=ADVANCED_FACE ( 'NONE', ( #6058 ), #4481, .T. ) ;
#1329=LINE ( 'NONE', #4992, #5381 ) ;
#1331=CARTESIAN_POINT ( 'NONE',  ( 4.666531114835057892, 48.52758949912974629, -2.680605614690282579 ) ) ;
#1342=VERTEX_POINT ( 'NONE', #7074 ) ;
#1343=CARTESIAN_POINT ( 'NONE',  ( -52.82691659388441252, 75.69008924411679118, 4.122156975067814422 ) ) ;
#1352=CARTESIAN_POINT ( 'NONE',  ( -18.69730990872651333, 70.57397863033268948, 14.11552877426516339 ) ) ;
#1354=CARTESIAN_POINT ( 'NONE',  ( 1.493523987181155643, 37.44802286055433171, -11.71834779115162561 ) ) ;
#1355=CARTESIAN_POINT ( 'NONE',  ( -5.928718717905509195, 56.37336801400213915, -14.01350978889703391 ) ) ;
#1362=CARTESIAN_POINT ( 'NONE',  ( -64.33684479406403511, 55.00260128198466703, -0.002143347410900310612 ) ) ;
#1363=VECTOR ( 'NONE', #5696, 1000.000000000000000 ) ;
#1364=B_SPLINE_CURVE_WITH_KNOTS ( 'NONE', 3,
 ( #3453, #5314, #3388, #9683, #6163, #8073, #11709, #5372, #569, #743, #4237, #8904, #7895, #11525, #6104, #9796, #9735, #1533, #4292, #1589, #7950, #4359, #11644, #10138, #17, #10863, #915, #802, #7293, #9249, #5669, #8184, #7473, #6448, #10974, #4473, #136, #3627, #6575, #1763, #3800, #4644, #10079, #1815, #5429, #8125, #5610, #1997, #10204, #1037, #1876, #5485, #10925, #11762, #11094, #2908, #8296, #3569, #6338, #1941, #982, #2736, #7240, #2673, #77, #9970, #9078, #856, #6393, #4528, #11820, #10022, #3738, #9134, #4585, #8240, #8352, #4704, #3686, #7351, #5547, #7405, #2786, #9190, #11032, #2842, #6511, #199, #2300, #4762, #11334, #10325, #9308, #6809, #3868, #8480, #256, #2062, #6755, #8417, #9428, #6632, #7643, #1099, #1218, #10261, #319, #7528, #7704, #5731, #3984, #380, #11275, #4046, #3143, #9366, #3086, #4948, #10384, #6871, #2965, #10436, #2238, #11150 ),
 .UNSPECIFIED., .F., .F.,
 ( 4, 2, 2, 2, 2, 2, 2, 2, 2, 2, 2, 2, 2, 2, 2, 2, 2, 2, 2, 2, 2, 2, 2, 2, 2, 2, 2, 2, 2, 2, 2, 2, 2, 2, 2, 2, 2, 2, 2, 2, 2, 2, 2, 2, 2, 2, 2, 2, 2, 2, 2, 2, 2, 2, 2, 2, 2, 2, 2, 2, 2, 4 ),
 ( 0.000000000000000000, 0.02499977550252127645, 0.04999988577693819519, 0.07499999605135511394, 0.09999999831535408279, 0.1250000005793530378, 0.1500000028441162425, 0.1750000051088794195, 0.1937500039558066045, 0.2031250033792701970, 0.2125000028027338173, 0.2218750022261974375, 0.2312500016496610300, 0.2500000004965882150, 0.2750000027613288545, 0.3000000050260694384, 0.3187500038730080032, 0.3281250032964772578, 0.3375000027199465125, 0.3468750021434158226, 0.3562500015668850772, 0.3750000004138236420, 0.4000000026785641705, 0.4250000049433046989, 0.4437500037902432082, 0.4531250032137125183, 0.4625000026371817730, 0.4718750020606510276, 0.4812500014841203377, 0.5000000003310588470, 0.5250000025957997085, 0.5500000048605405700, 0.5687500037074788573, 0.5781250031309480564, 0.5875000025544172555, 0.5968750019778864546, 0.6062500014013556537, 0.6250000002482940520, 0.6500000025128280789, 0.6750000047773621059, 0.6937500036244039769, 0.7031250030479249125, 0.7125000024714458480, 0.7218750018949667835, 0.7312500013184877190, 0.7500000001655295900, 0.7750000023794885173, 0.8000000045934475557, 0.8187500034657768655, 0.8281250029019414649, 0.8375000023381060643, 0.8468750017742707747, 0.8562500012104353742, 0.8750000000827646840, 0.8937502654913498379, 0.9031253981956424148, 0.9125005308999349918, 0.9218756636042275687, 0.9312507963085201457, 0.9500010617171052996, 0.9750005308585526498, 1.000000000000000000 ),
 .UNSPECIFIED. ) ;
#1369=CARTESIAN_POINT ( 'NONE',  ( -43.58294393097721553, 55.68691547946620801, -6.980998355533345467 ) ) ;
#1370=ORIENTED_EDGE ( 'NONE', *, *, #2171, .F. ) ;
#1371=CARTESIAN_POINT ( 'NONE',  ( -29.54809237377008202, 34.60091625530366599, 5.109976345715927515 ) ) ;
#1373=LINE ( 'NONE', #11304, #11545 ) ;
#1383=DIRECTION ( 'NONE',  ( 1.000000000000000000, 0.000000000000000000, 0.000000000000000000 ) ) ;
#1384=CARTESIAN_POINT ( 'NONE',  ( -19.32947785509334082, 63.04547287423799418, 19.42212676744230393 ) ) ;
#1385=DIRECTION ( 'NONE',  ( 1.000000000000000000, 6.033820786006286457E-17, -0.000000000000000000 ) ) ;
#1392=CARTESIAN_POINT ( 'NONE',  ( -52.42856357389445066, 59.99999999999997158, -5.034386850915387018E-15 ) ) ;
#1394=CARTESIAN_POINT ( 'NONE',  ( -45.89008546996493720, 61.09306511264237827, -3.515648168893299896 ) ) ;
#1395=DIRECTION ( 'NONE',  ( 1.000000000000000000, 6.033820786006286457E-17, 0.000000000000000000 ) ) ;
#1404=CARTESIAN_POINT ( 'NONE',  ( -1.240525345857069306, 54.99835318325028055, 0.02617781847627572225 ) ) ;
#1412=CARTESIAN_POINT ( 'NONE',  ( -42.33720994522852266, 55.00043528610386545, -21.02753041772728437 ) ) ;
#1413=ORIENTED_EDGE ( 'NONE', *, *, #6593, .F. ) ;
#1414=CARTESIAN_POINT ( 'NONE',  ( 6.173066176615439105, 34.30768362678504957, 4.109395208432498947 ) ) ;
#1415=CARTESIAN_POINT ( 'NONE',  ( -24.79373960380069164, 53.16908519469900085, 14.01800865919465799 ) ) ;
#1424=CARTESIAN_POINT ( 'NONE',  ( -48.44321661921154032, 60.60981481080942501, -4.313990038473558108 ) ) ;
#1426=CARTESIAN_POINT ( 'NONE',  ( -28.36397722366938012, 36.00052710555507218, 8.986026874162561739 ) ) ;
#1427=CARTESIAN_POINT ( 'NONE',  ( 14.47760468889531182, 57.74566952947367326, 20.98118467575540436 ) ) ;
#1437=CARTESIAN_POINT ( 'NONE',  ( -11.52239577449127061, 75.97627689174807131, -2.745668057393931161 ) ) ;
#1442=VERTEX_POINT ( 'NONE', #4653 ) ;
#1445=DIRECTION ( 'NONE',  ( 9.813077866773612233E-16, -1.000000000000000000, -0.000000000000000000 ) ) ;
#1449=CARTESIAN_POINT ( 'NONE',  ( -50.16689083095988622, 61.89286798645840548, 1.372268717346541989 ) ) ;
#1451=ADVANCED_FACE ( 'NONE', ( #8251 ), #2684, .T. ) ;
#1464=CARTESIAN_POINT ( 'NONE',  ( -16.87154951642690648, 55.00301719933347044, 0.003379411846644060982 ) ) ;
#1467=ORIENTED_EDGE ( 'NONE', *, *, #8813, .F. ) ;
#1469=CARTESIAN_POINT ( 'NONE',  ( -36.14426256656389569, 36.63180902967581432, -10.58010824564746599 ) ) ;
#1471=CARTESIAN_POINT ( 'NONE',  ( -7.548092367965108629, 65.81078796322651669, -18.03704516092939869 ) ) ;
#1472=CARTESIAN_POINT ( 'NONE',  ( -31.00186844413243392, 42.04798375885678752, 5.364520326994415278 ) ) ;
#1478=DIRECTION ( 'NONE',  ( 1.000000000000000000, 6.033820786006286457E-17, -0.000000000000000000 ) ) ;
#1482=DIRECTION ( 'NONE',  ( -9.813077866773612233E-16, 1.000000000000000000, 0.000000000000000000 ) ) ;
#1483=CARTESIAN_POINT ( 'NONE',  ( -19.66652697884454781, 59.95698360088004364, 4.957362171560429687 ) ) ;
#1486=CARTESIAN_POINT ( 'NONE',  ( -42.96936073659074395, 63.99245613053683712, -19.01383356661934343 ) ) ;
#1497=CARTESIAN_POINT ( 'NONE',  ( 6.636022776496402820, 34.00797225689733239, 1.031222807066483504 ) ) ;
#1500=DIRECTION ( 'NONE',  ( 0.000000000000000000, 1.000000000000000000, 0.000000000000000000 ) ) ;
#1508=CARTESIAN_POINT ( 'NONE',  ( -28.58294521375118791, 48.28461196395628718, 2.037989642863114348 ) ) ;
#1518=CARTESIAN_POINT ( 'NONE',  ( -18.61890672186335749, 55.00248007087589741, 0.008241009575747904742 ) ) ;
#1523=ORIENTED_EDGE ( 'NONE', *, *, #3095, .T. ) ;
#1526=CARTESIAN_POINT ( 'NONE',  ( -31.54809236465146682, 34.60179423563022283, 5.109615027512485419 ) ) ;
#1528=CARTESIAN_POINT ( 'NONE',  ( -47.85572436634423354, 73.33185325676623734, -10.56518764769322516 ) ) ;
#1529=CARTESIAN_POINT ( 'NONE',  ( -17.59538538452048684, 67.42122968706608788, 6.631564624215115167 ) ) ;
#1533=CARTESIAN_POINT ( 'NONE',  ( 6.636022776496402820, 34.00797225689733239, 1.031222807066483504 ) ) ;
#1534=ORIENTED_EDGE ( 'NONE', *, *, #3310, .T. ) ;
#1538=CARTESIAN_POINT ( 'NONE',  ( -53.50022385974906314, 61.89434742217085272, 1.372896053409885520 ) ) ;
#1540=CARTESIAN_POINT ( 'NONE',  ( -57.27472358375123207, 61.14040963541170015, 20.20590277145669234 ) ) ;
#1551=CARTESIAN_POINT ( 'NONE',  ( -13.14429486149114013, 76.02373996650987920, 2.745652855075435994 ) ) ;
#1556=CARTESIAN_POINT ( 'NONE',  ( -58.64797208933948269, 57.51009499518404056, 4.336531854824778875 ) ) ;
#1559=CARTESIAN_POINT ( 'NONE',  ( -22.50647595179652072, 59.12487335784310005, 20.69694904210189179 ) ) ;
#1567=ORIENTED_EDGE ( 'NONE', *, *, #9736, .T. ) ;
#1568=CARTESIAN_POINT ( 'NONE',  ( -57.16684244878135246, 56.37008073134157371, 6.893775596464392308 ) ) ;
#1577=DIRECTION ( 'NONE',  ( -1.000000000000000000, -6.033820786006286457E-17, 0.000000000000000000 ) ) ;
#1578=CARTESIAN_POINT ( 'NONE',  ( 18.24053854380704820, 55.00849189285069230, 0.02483751907359685318 ) ) ;
#1584=CARTESIAN_POINT ( 'NONE',  ( -51.60828739328132997, 76.01535744515140891, 2.059423361852914969 ) ) ;
#1585=CARTESIAN_POINT ( 'NONE',  ( -52.59538850930821496, 69.01351387254386793, 1.373364761778438581 ) ) ;
#1589=CARTESIAN_POINT ( 'NONE',  ( 5.737308841168996310, 34.06700459503902323, -2.059191599423306318 ) ) ;
#1593=CARTESIAN_POINT ( 'NONE',  ( 23.81438878217834088, 59.74505718300422075, 1.610512999816130497 ) ) ;
#1594=CARTESIAN_POINT ( 'NONE',  ( -67.10978172608912473, 49.39091922923409328, 4.313686075943445886 ) ) ;
#1595=ORIENTED_EDGE ( 'NONE', *, *, #7678, .F. ) ;
#1596=CARTESIAN_POINT ( 'NONE',  ( -7.737413764666613680, 68.33402667507452577, -16.24506794676610610 ) ) ;
#1606=CARTESIAN_POINT ( 'NONE',  ( -37.18898618307433424, 44.43582214169357769, -18.32873044267784479 ) ) ;
#1612=CARTESIAN_POINT ( 'NONE',  ( 8.623112943508827399, 51.69526317675230587, 3.766397512801251235 ) ) ;
#1620=CARTESIAN_POINT ( 'NONE',  ( -42.00013555804697774, 57.68060557487371653, -6.472410377448052365 ) ) ;
#1626=VERTEX_POINT ( 'NONE', #2920 ) ;
#1632=CARTESIAN_POINT ( 'NONE',  ( -6.952240055115057160, 55.00666461818682507, -0.005444984560454538616 ) ) ;
#1635=CARTESIAN_POINT ( 'NONE',  ( -20.51396975634441944, 55.33168391584075607, 4.991693283627284039 ) ) ;
#1639=CARTESIAN_POINT ( 'NONE',  ( -50.18900491406688502, 75.97955728750814330, -2.745941717788443537 ) ) ;
#1647=ORIENTED_EDGE ( 'NONE', *, *, #1808, .F. ) ;
#1649=CARTESIAN_POINT ( 'NONE',  ( 25.76190476190475565, 59.99999999999995026, 0.000000000000000000 ) ) ;
#1650=CARTESIAN_POINT ( 'NONE',  ( -8.909737369126560225, 55.00301576531230552, -0.005174452243964258909 ) ) ;
#1652=CARTESIAN_POINT ( 'NONE',  ( -57.82750524721426189, 59.10997802641301035, 20.69196764327204008 ) ) ;
#1653=VECTOR ( 'NONE', #2471, 1000.000000000000000 ) ;
#1654=CARTESIAN_POINT ( 'NONE',  ( -34.72515708538001888, 34.82355399787605421, -6.128525890628534256 ) ) ;
#1663=CARTESIAN_POINT ( 'NONE',  ( -63.06671435217206323, 41.62111505249539078, 16.30162306856191989 ) ) ;
#1667=CARTESIAN_POINT ( 'NONE',  ( -61.36749305124384080, 55.33290285919624552, 4.999731327536861336 ) ) ;
#1671=CARTESIAN_POINT ( 'NONE',  ( 7.462649519108526697, 51.02641210518733317, 3.052499146972269983 ) ) ;
#1673=CARTESIAN_POINT ( 'NONE',  ( 53.00000000000000000, 51.46446609406726935, -3.535533905932738197 ) ) ;
#1675=VERTEX_POINT ( 'NONE', #9204 ) ;
#1679=CARTESIAN_POINT ( 'NONE',  ( -11.20624054502364864, 68.97545947489571461, -1.830994258430044930 ) ) ;
#1695=CARTESIAN_POINT ( 'NONE',  ( -27.38106182849360337, 55.00820573016070369, -0.003135496005600075728 ) ) ;
#1700=CARTESIAN_POINT ( 'NONE',  ( -11.37681534325029098, 59.99999999999997868, -0.1654421410166476147 ) ) ;
#1703=CARTESIAN_POINT ( 'NONE',  ( -20.66281120459677823, 63.04561409439726560, 19.42247919112690013 ) ) ;
#1712=CARTESIAN_POINT ( 'NONE',  ( 7.290226732917977515, 50.00000000000001421, 0.1647554015558948537 ) ) ;
#1713=CARTESIAN_POINT ( 'NONE',  ( -4.426057251632187217, 54.99526716342594312, -0.01575941339944971972 ) ) ;
#1716=CARTESIAN_POINT ( 'NONE',  ( 3.030639393851187524, 35.98666035303370592, -8.992230872156422805 ) ) ;
#1717=CARTESIAN_POINT ( 'NONE',  ( -31.26269038945179446, 34.87416470039633509, 6.107602927758665423 ) ) ;
#1727=DIRECTION ( 'NONE',  ( 0.000000000000000000, 1.000000000000000000, 0.000000000000000000 ) ) ;
#1741=CARTESIAN_POINT ( 'NONE',  ( -1.457434152866251775, 54.34000425242091126, -4.958991060964934583 ) ) ;
#1742=CARTESIAN_POINT ( 'NONE',  ( -25.20616590903865628, 46.41268961681102212, 11.17697077816622020 ) ) ;
#1753=CARTESIAN_POINT ( 'NONE',  ( -26.50353529629213867, 55.00548998525069067, -0.001986402032320984824 ) ) ;
#1755=CARTESIAN_POINT ( 'NONE',  ( -22.46041777029512332, 53.70875712283432790, 4.841299448188346233 ) ) ;
#1759=CARTESIAN_POINT ( 'NONE',  ( -60.03167053577592327, 56.03207409872247524, 20.99365918962282862 ) ) ;
#1763=CARTESIAN_POINT ( 'NONE',  ( -7.662811188708723797, 69.86483622371564195, -14.86557385339502169 ) ) ;
#1764=( NAMED_UNIT ( * ) PLANE_ANGLE_UNIT ( ) SI_UNIT ( $, .RADIAN. ) );
#1769=CARTESIAN_POINT ( 'NONE',  ( -65.16650212331052217, 51.09201045536845953, 5.853437054489593727 ) ) ;
#1771=CARTESIAN_POINT ( 'NONE',  ( -59.88037020503378471, 51.91452991566635689, 20.80113349088246011 ) ) ;
#1772=CARTESIAN_POINT ( 'NONE',  ( -36.85572911278101316, 38.22258139949027367, -12.89445763391127464 ) ) ;
#1776=VERTEX_POINT ( 'NONE', #10450 ) ;
#1778=CARTESIAN_POINT ( 'NONE',  ( -46.82983832526868184, 55.00115022211477367, -0.002242098181359713800 ) ) ;
#1779=CARTESIAN_POINT ( 'NONE',  ( -57.84573968844613034, 55.33154914686375037, 4.999987675084161864 ) ) ;
#1782=CARTESIAN_POINT ( 'NONE',  ( -70.31421248054985540, 50.03279511399161095, 0.6584628854196864500 ) ) ;
#1791=CARTESIAN_POINT ( 'NONE',  ( 36.99999999999999289, 64.99999999999998579, 0.000000000000000000 ) ) ;
#1794=CARTESIAN_POINT ( 'NONE',  ( 5.788533022989986065, 41.13062614362130631, -2.057011258941260134 ) ) ;
#1803=CARTESIAN_POINT ( 'NONE',  ( -64.24754237443872285, 55.03769318549124279, -0.006317726105072558364 ) ) ;
#1806=CARTESIAN_POINT ( 'NONE',  ( -10.01312846213127905, 59.83883587255158432, -1.300640683813629295 ) ) ;
#1808=EDGE_CURVE ( 'NONE', #3357, #11411, #2251, .T. ) ;
#1809=CARTESIAN_POINT ( 'NONE',  ( -69.52691976458234535, 34.01892180236649921, 2.749684864678113794 ) ) ;
#1811=CARTESIAN_POINT ( 'NONE',  ( 4.636023424558444184, 34.00634798409771520, 1.031279783234476222 ) ) ;
#1815=CARTESIAN_POINT ( 'NONE',  ( -10.81092923698156838, 75.47407628921179423, -5.508885182882011122 ) ) ;
#1817=VERTEX_POINT ( 'NONE', #216 ) ;
#1820=CARTESIAN_POINT ( 'NONE',  ( -11.82983844552040686, 55.00192051767528767, -0.001631283583225531103 ) ) ;
#1823=CARTESIAN_POINT ( 'NONE',  ( -31.07074709816078695, 34.08442161144734683, 2.058417023654369071 ) ) ;
#1824=EDGE_CURVE ( 'NONE', #7013, #10196, #8656, .T. ) ;
#1825=CARTESIAN_POINT ( 'NONE',  ( -31.54809236465146682, 34.60179423563022283, 5.109615027512485419 ) ) ;
#1833=CARTESIAN_POINT ( 'NONE',  ( -22.61890542003328619, 55.00133982146918044, 0.005189527613788253065 ) ) ;
#1834=CARTESIAN_POINT ( 'NONE',  ( -32.95459766285684822, 50.50504115442574005, -2.214447714617367335 ) ) ;
#1842=LINE ( 'NONE', #8146, #4176 ) ;
#1844=CARTESIAN_POINT ( 'NONE',  ( 13.68354351360180132, 55.65895967216258811, 4.967044982674917009 ) ) ;
#1851=DIRECTION ( 'NONE',  ( -1.000000000000000000, -0.000000000000000000, -0.000000000000000000 ) ) ;
#1853=CARTESIAN_POINT ( 'NONE',  ( 8.404614611173400363, 41.52310116625425707, 4.095790913453249082 ) ) ;
#1859=EDGE_LOOP ( 'NONE', ( #8569, #2807, #7885, #8102 ) ) ;
#1864=CARTESIAN_POINT ( 'NONE',  ( -62.09272923114016862, 55.00758854939876841, -0.01093042735399621553 ) ) ;
#1867=CARTESIAN_POINT ( 'NONE',  ( -26.34413835852909713, 51.02730822250849485, 3.053792540648594844 ) ) ;
#1872=CARTESIAN_POINT ( 'NONE',  ( 19.14436220527237253, 71.77763100192429135, 12.89423484158165500 ) ) ;
#1876=CARTESIAN_POINT ( 'NONE',  ( -17.00387655282055377, 69.86881140706658755, 14.86941770366936311 ) ) ;
#1880=CARTESIAN_POINT ( 'NONE',  ( -7.706467115899972242, 56.60995633697762486, -4.745024238781081927 ) ) ;
#1882=CARTESIAN_POINT ( 'NONE',  ( 0.8268573817076104726, 37.44832105976551873, -11.71822709476406210 ) ) ;
#1884=CARTESIAN_POINT ( 'NONE',  ( -29.33720989395294509, 35.57257717978642830, 8.046635596291469739 ) ) ;
#1886=CARTESIAN_POINT ( 'NONE',  ( -25.18906244525692983, 49.50751464484449826, 20.43480895838654376 ) ) ;
#1894=CARTESIAN_POINT ( 'NONE',  ( -20.57640403573022780, 55.00362648708293989, 0.004766381080466141652 ) ) ;
#1896=CARTESIAN_POINT ( 'NONE',  ( -54.93158096975896143, 57.64487218557030701, 4.246342238008629977 ) ) ;
#1898=CYLINDRICAL_SURFACE ( 'NONE', #11310, 4.999999999999984013 ) ;
#1901=CARTESIAN_POINT ( 'NONE',  ( -7.070747353360942178, 68.33360022464046324, -16.24461469319379603 ) ) ;
#1904=CARTESIAN_POINT ( 'NONE',  ( -29.87222872871134527, 51.02501382459326607, 3.050615963077655035 ) ) ;
#1909=ORIENTED_EDGE ( 'NONE', *, *, #869, .F. ) ;
#1911=VERTEX_POINT ( 'NONE', #2699 ) ;
#1912=CARTESIAN_POINT ( 'NONE',  ( -6.515206263428001243, 58.30176811177454255, -3.769010736591787314 ) ) ;
#1913=CARTESIAN_POINT ( 'NONE',  ( -18.99814003679748708, 60.36334191107018654, 12.94714326548398731 ) ) ;
#1926=CARTESIAN_POINT ( 'NONE',  ( -35.42605725946955886, 54.98265126924874124, -0.01969512534468634626 ) ) ;
#1935=CARTESIAN_POINT ( 'NONE',  ( -9.070746587277097817, 68.33487957594263662, -16.24597445391072270 ) ) ;
#1939=EDGE_LOOP ( 'NONE', ( #5728, #5478, #8347, #5802 ) ) ;
#1941=CARTESIAN_POINT ( 'NONE',  ( -22.47759590436300314, 52.25445647903773505, 21.02373912143526979 ) ) ;
#1943=CARTESIAN_POINT ( 'NONE',  ( -36.47762819585614835, 42.07544065584382764, -16.80749884933775462 ) ) ;
#1947=CARTESIAN_POINT ( 'NONE',  ( 63.00000000000000000, 55.00000000000000000, 0.000000000000000000 ) ) ;
#1948=VERTEX_POINT ( 'NONE', #6364 ) ;
#1949=CARTESIAN_POINT ( 'NONE',  ( -19.11869220366278199, 65.80735234221702967, 18.02962863481653955 ) ) ;
#1950=CARTESIAN_POINT ( 'NONE',  ( -57.50627882723209439, 66.73110044028416610, 17.54296274220338958 ) ) ;
#1953=DIRECTION ( 'NONE',  ( 1.000000000000000000, 6.033820786006286457E-17, -0.000000000000000000 ) ) ;
#1957=CARTESIAN_POINT ( 'NONE',  ( -32.53821616509017645, 54.99747915939720144, 0.0007716475280872252956 ) ) ;
#1958=CARTESIAN_POINT ( 'NONE',  ( -51.62174940093352404, 59.49509050522294729, 2.214026401944775735 ) ) ;
#1960=LINE ( 'NONE', #9388, #7831 ) ;
#1962=CARTESIAN_POINT ( 'NONE',  ( -60.16384031450671444, 57.73999876476588611, 13.79403801089012660 ) ) ;
#1966=CARTESIAN_POINT ( 'NONE',  ( -32.21076886968869246, 50.12793110694000376, 1.301955266658537003 ) ) ;
#1974=CARTESIAN_POINT ( 'NONE',  ( -59.25590502003253590, 53.62714168963238848, 13.95829701047152405 ) ) ;
#1982=CARTESIAN_POINT ( 'NONE',  ( -33.95704062082862862, 50.00000000000001421, -0.1649495599488684516 ) ) ;
#1985=CARTESIAN_POINT ( 'NONE',  ( -7.291280311133348846, 60.19918483626972971, -4.712039246562317096 ) ) ;
#1987=FACE_OUTER_BOUND ( 'NONE', #8654, .T. ) ;
#1992=CARTESIAN_POINT ( 'NONE',  ( 36.99999999999999289, 55.00000000000000000, 0.000000000000000000 ) ) ;
#1994=CARTESIAN_POINT ( 'NONE',  ( -5.608280846031337141, 57.05942937149918492, -21.01412426850803783 ) ) ;
#1997=CARTESIAN_POINT ( 'NONE',  ( -15.27494751580540111, 73.62981360231496808, 9.945832149094092856 ) ) ;
#1998=( LENGTH_UNIT ( ) NAMED_UNIT ( * ) SI_UNIT ( .MILLI., .METRE. ) );
#1999=CARTESIAN_POINT ( 'NONE',  ( -59.00490307935969270, 55.00061426705308065, 21.02882928537637497 ) ) ;
#2000=EDGE_LOOP ( 'NONE', ( #11386, #9598, #3097, #7550 ) ) ;
#2002=CARTESIAN_POINT ( 'NONE',  ( -6.152294610831279265, 55.33101663292276129, -5.000007508712183579 ) ) ;
#2003=CARTESIAN_POINT ( 'NONE',  ( -7.337209909475700620, 63.04728967918421745, -19.42673836724018699 ) ) ;
#2005=CARTESIAN_POINT ( 'NONE',  ( -43.32947769439600449, 63.04458385766601936, -19.42270034872903750 ) ) ;
#2006=CARTESIAN_POINT ( 'NONE',  ( 14.12709322831273795, 56.83099522254385505, 13.98200332532292123 ) ) ;
#2013=CARTESIAN_POINT ( 'NONE',  ( -45.66879787574058724, 54.99910181478063009, 0.001600114446596862059 ) ) ;
#2014=CARTESIAN_POINT ( 'NONE',  ( -48.51431238046460237, 59.99999999999936051, -0.3319244779807851708 ) ) ;
#2016=VECTOR ( 'NONE', #1478, 1000.000000000000000 ) ;
#2017=DIRECTION ( 'NONE',  ( 0.000000000000000000, 1.000000000000000000, 0.000000000000000000 ) ) ;
#2018=CARTESIAN_POINT ( 'NONE',  ( -4.109914231205427981, 53.16120966094572964, -6.833699982310251109 ) ) ;
#2020=CARTESIAN_POINT ( 'NONE',  ( 2.274842917244503937, 38.70728229458904934, -13.38060881307704975 ) ) ;
#2021=CARTESIAN_POINT ( 'NONE',  ( 47.00000000000000000, 51.46446609406726935, 3.535533905932731091 ) ) ;
#2022=CARTESIAN_POINT ( 'NONE',  ( -30.65099889004999412, 50.66178966001721307, 2.507330033107963985 ) ) ;
#2029=EDGE_LOOP ( 'NONE', ( #3742, #691, #10930, #8070 ) ) ;
#2031=CARTESIAN_POINT ( 'NONE',  ( -29.21146697695694527, 41.39918523644610104, 3.407148991788945924 ) ) ;
#2037=ORIENTED_EDGE ( 'NONE', *, *, #899, .F. ) ;
#2043=CARTESIAN_POINT ( 'NONE',  ( -34.54441260842353500, 50.04071390848193346, -0.6575957411896632410 ) ) ;
#2045=CARTESIAN_POINT ( 'NONE',  ( 7.000139726508040283, 47.98854375967137287, -0.0002567025502792563349 ) ) ;
#2055=CARTESIAN_POINT ( 'NONE',  ( -20.73741325422386339, 64.90628579765783002, 18.53688757488948369 ) ) ;
#2058=EDGE_CURVE ( 'NONE', #1342, #678, #10330, .T. ) ;
#2062=CARTESIAN_POINT ( 'NONE',  ( -51.69727455458300369, 74.78870212167194609, 7.080596778485133136 ) ) ;
#2069=CARTESIAN_POINT ( 'NONE',  ( -31.96936060593014162, 33.99278688086445044, -1.031647977713077813 ) ) ;
#2070=CARTESIAN_POINT ( 'NONE',  ( -67.17448730496187181, 36.66801277209461318, 10.55271442276269944 ) ) ;
#2076=CARTESIAN_POINT ( 'NONE',  ( -65.49460043985243374, 54.99687722424931025, 0.003115495885130020737 ) ) ;
#2077=DIRECTION ( 'NONE',  ( 1.000000000000000000, 6.033820786006286457E-17, 0.000000000000000000 ) ) ;
#2079=DIRECTION ( 'NONE',  ( 1.000000000000000000, 6.033820786006286457E-17, 0.000000000000000000 ) ) ;
#2080=CARTESIAN_POINT ( 'NONE',  ( 18.44333507102063763, 60.58560716114385514, 4.289589058474648553 ) ) ;
#2083=CARTESIAN_POINT ( 'NONE',  ( 5.737308841168996310, 34.06700459503902323, -2.059191599423306318 ) ) ;
#2095=CARTESIAN_POINT ( 'NONE',  ( -56.92857623826265012, 59.09574567893412222, 13.47676509801295452 ) ) ;
#2105=CARTESIAN_POINT ( 'NONE',  ( -41.15537497174283743, 53.39487353770535805, -4.746796348801736620 ) ) ;
#2106=CARTESIAN_POINT ( 'NONE',  ( -3.500223734511656026, 56.37227171202499676, -6.892880562731030558 ) ) ;
#2107=AXIS2_PLACEMENT_3D ( 'NONE', #1947, #11156, #10084 ) ;
#2115=CARTESIAN_POINT ( 'NONE',  ( -28.94161417925737823, 38.68453375511723635, 13.40299329694203578 ) ) ;
#2127=CARTESIAN_POINT ( 'NONE',  ( 3.180458482999132919, 49.99999999999981526, -0.3308461596649949210 ) ) ;
#2130=CARTESIAN_POINT ( 'NONE',  ( 12.81090570363319436, 49.50804083114603316, 20.43325688243531602 ) ) ;
#2132=CARTESIAN_POINT ( 'NONE',  ( -56.32961277634869646, 69.86611656190129338, 14.86520567151240080 ) ) ;
#2139=VERTEX_POINT ( 'NONE', #4891 ) ;
#2145=CARTESIAN_POINT ( 'NONE',  ( -63.66377439455398246, 49.63604620300440473, 12.94636655892279009 ) ) ;
#2147=CARTESIAN_POINT ( 'NONE',  ( -23.18906244097991021, 49.50939288222085821, 20.43027456479002879 ) ) ;
#2157=CARTESIAN_POINT ( 'NONE',  ( -54.29700862423385388, 64.41868735558820447, 10.39170421311061254 ) ) ;
#2165=CARTESIAN_POINT ( 'NONE',  ( -38.81824253360387189, 51.69821110756454630, -3.768992944301960968 ) ) ;
#2167=CARTESIAN_POINT ( 'NONE',  ( 24.10985792112495218, 61.79436671605726161, 1.822573681661085354 ) ) ;
#2171=EDGE_CURVE ( 'NONE', #9767, #567, #3050, .T. ) ;
#2175=CARTESIAN_POINT ( 'NONE',  ( -55.45210586135002728, 71.88485191958531573, 12.52183031059725771 ) ) ;
#2185=CARTESIAN_POINT ( 'NONE',  ( -25.18906244525692983, 49.50751464484449826, 20.43480895838654376 ) ) ;
#2187=CARTESIAN_POINT ( 'NONE',  ( -63.17697253202724283, 43.28183360602782415, 17.55497741318475491 ) ) ;
#2188=CARTESIAN_POINT ( 'NONE',  ( 3.121866368482561160, 41.13189203504037295, -2.057008360219124032 ) ) ;
#2199=( GEOMETRIC_REPRESENTATION_CONTEXT ( 3 ) GLOBAL_UNCERTAINTY_ASSIGNED_CONTEXT ( ( #3996 ) ) GLOBAL_UNIT_ASSIGNED_CONTEXT ( ( #1998, #1764, #10023 ) ) REPRESENTATION_CONTEXT ( 'NONE', 'WORKASPACE' ) );
#2203=CARTESIAN_POINT ( 'NONE',  ( -70.67038125215350419, 40.99581249687635420, 0.003422455583789344152 ) ) ;
#2205=CARTESIAN_POINT ( 'NONE',  ( -42.66281101964754896, 63.04450918361814615, -19.42252581123130639 ) ) ;
#2217=CARTESIAN_POINT ( 'NONE',  ( -58.66904817996947941, 55.00018295349421749, 14.02051935868267307 ) ) ;
#2228=CARTESIAN_POINT ( 'NONE',  ( 7.291299706434547723, 48.00851142473923971, 0.3439031866554066452 ) ) ;
#2235=CARTESIAN_POINT ( 'NONE',  ( -34.72515708538001888, 34.82355399787605421, -6.128525890628534256 ) ) ;
#2238=CARTESIAN_POINT ( 'NONE',  ( -67.52720549794999272, 34.02364409886038743, 2.748840581154547102 ) ) ;
#2245=CARTESIAN_POINT ( 'NONE',  ( -21.63602683877659771, 62.08561388645346568, 19.80191166437241179 ) ) ;
#2247=CARTESIAN_POINT ( 'NONE',  ( -15.18898619350627754, 75.43339460814846120, 5.491620057114340092 ) ) ;
#2248=CARTESIAN_POINT ( 'NONE',  ( -1.460406270097956538, 46.38242329338708458, -11.20688125615216890 ) ) ;
#2251=LINE ( 'NONE', #10338, #8612 ) ;
#2254=CARTESIAN_POINT ( 'NONE',  ( -60.23628175600274659, 55.00363048015435652, 0.01172028139553065243 ) ) ;
#2259=CARTESIAN_POINT ( 'NONE',  ( -41.83355676456199745, 53.63003671930656679, -6.894939712124843467 ) ) ;
#2261=CARTESIAN_POINT ( 'NONE',  ( -38.60828084422895046, 48.85949782923615459, -20.20603288453101243 ) ) ;
#2263=LINE ( 'NONE', #284, #458 ) ;
#2266=LINE ( 'NONE', #5940, #2293 ) ;
#2272=CARTESIAN_POINT ( 'NONE',  ( 5.451907626115248817, 34.19820075889870026, -3.085388827037094828 ) ) ;
#2283=DIRECTION ( 'NONE',  ( 1.000000000000000000, 6.033820786006286457E-17, -0.000000000000000000 ) ) ;
#2289=CARTESIAN_POINT ( 'NONE',  ( -58.33319328058090036, 54.99975163993536142, 7.012209431990541475 ) ) ;
#2293=VECTOR ( 'NONE', #9580, 1000.000000000000000 ) ;
#2297=ORIENTED_EDGE ( 'NONE', *, *, #291, .F. ) ;
#2300=CARTESIAN_POINT ( 'NONE',  ( -42.96936073659074395, 63.99245613053683712, -19.01383356661934343 ) ) ;
#2306=CARTESIAN_POINT ( 'NONE',  ( -30.36397657560652874, 35.99904827701746513, 8.986701095552454888 ) ) ;
#2308=CARTESIAN_POINT ( 'NONE',  ( 3.262586490554605145, 34.88822117712475546, -6.102536506291977858 ) ) ;
#2309=CARTESIAN_POINT ( 'NONE',  ( -44.41060717808029068, 59.06754546170965625, -13.40628650917997433 ) ) ;
#2310=DIRECTION ( 'NONE',  ( 1.000000000000000000, 6.033820786006286457E-17, 0.000000000000000000 ) ) ;
#2323=CARTESIAN_POINT ( 'NONE',  ( -46.49982872022311398, 58.90684247826047937, -5.852054447348608690 ) ) ;
#2325=CARTESIAN_POINT ( 'NONE',  ( -21.05849041552747281, 57.05917194494736577, 20.98221040122819403 ) ) ;
#2327=CLOSED_SHELL ( 'NONE', ( #8712, #5217, #8658, #10847, #4602, #10093, #4565, #4457, #1451, #1323, #9407, #808, #3976, #7463, #639, #2403, #8067, #3823, #11041, #3447, #3010, #7533, #266, #4848, #3457, #5436, #5812, #10805, #7204, #5209, #7295, #8665, #374 ) ) ;
#2328=CARTESIAN_POINT ( 'NONE',  ( 19.85574934264614910, 73.36821619702706698, 10.58005382006121131 ) ) ;
#2339=CARTESIAN_POINT ( 'NONE',  ( 10.18903847268274276, 38.19250115101311849, 12.92455934260550521 ) ) ;
#2340=DIRECTION ( 'NONE',  ( 0.000000000000000000, 1.000000000000000000, 0.000000000000000000 ) ) ;
#2343=DIRECTION ( 'NONE',  ( -0.7071067811865519026, 8.659560562354878624E-17, -0.7071067811865431318 ) ) ;
#2350=CARTESIAN_POINT ( 'NONE',  ( -26.24915659512696919, 49.55079243168071912, 4.477208298354541149 ) ) ;
#2360=CARTESIAN_POINT ( 'NONE',  ( 3.236198281082953265, 55.01300725603349662, 0.01475152511819301064 ) ) ;
#2365=CARTESIAN_POINT ( 'NONE',  ( -20.45202553191040806, 65.80759480864719535, 18.03021102644938267 ) ) ;
#2366=VERTEX_POINT ( 'NONE', #251 ) ;
#2367=CARTESIAN_POINT ( 'NONE',  ( 22.14421007127711860, 75.43322280825043435, 5.492045153080157505 ) ) ;
#2368=CARTESIAN_POINT ( 'NONE',  ( -11.73803863240502388, 67.39634740869848883, -6.621068033304872813 ) ) ;
#2370=CARTESIAN_POINT ( 'NONE',  ( -21.31755583740063287, 57.50727203353319794, 4.338243946322617894 ) ) ;
#2376=CARTESIAN_POINT ( 'NONE',  ( -17.91582325644631268, 61.21604956945397902, 3.318707400256076134 ) ) ;
#2378=CARTESIAN_POINT ( 'NONE',  ( -26.94161418247137263, 38.68192823000178038, 13.40559829713685502 ) ) ;
#2379=CARTESIAN_POINT ( 'NONE',  ( 4.329456757236127551, 33.97246960341611555, -0.0004353087921988608999 ) ) ;
#2389=CARTESIAN_POINT ( 'NONE',  ( -6.214759040711413718, 65.81103152010582846, -18.03762937187994453 ) ) ;
#2403=ADVANCED_FACE ( 'NONE', ( #3794 ), #10198, .T. ) ;
#2404=CARTESIAN_POINT ( 'NONE',  ( -64.55652465667151318, 48.91659104782370804, 3.512441407871431664 ) ) ;
#2407=VECTOR ( 'NONE', #8603, 1000.000000000000227 ) ;
#2413=ADVANCED_BREP_SHAPE_REPRESENTATION ( '', ( #684, #4738 ), #7754 ) ;
#2418=CARTESIAN_POINT ( 'NONE',  ( 5.576336621552477446, 55.00935349608988645, 0.004200982382114487428 ) ) ;
#2425=CARTESIAN_POINT ( 'NONE',  ( -13.52239577877046095, 75.98118489547775312, -2.745668029642679642 ) ) ;
#2428=CARTESIAN_POINT ( 'NONE',  ( -28.27494751366310766, 38.68366524674433293, 13.40386163033813460 ) ) ;
#2429=CARTESIAN_POINT ( 'NONE',  ( -7.369671227794407642, 59.71994724795483478, -13.19184786971608858 ) ) ;
#2431=CIRCLE ( 'NONE', #6849, 4.999999999999997335 ) ;
#2441=CARTESIAN_POINT ( 'NONE',  ( -56.12525174590880539, 60.62665842901460422, 4.172128455226769006 ) ) ;
#2444=CARTESIAN_POINT ( 'NONE',  ( 18.14435054219095633, 65.56481479683655778, 18.33023711405786926 ) ) ;
#2445=CARTESIAN_POINT ( 'NONE',  ( 8.189038476963473201, 38.19597440261895827, 12.92108669627241646 ) ) ;
#2452=CARTESIAN_POINT ( 'NONE',  ( -67.56971494453328830, 50.00000002031717372, -0.0004507456344833478141 ) ) ;
#2454=CARTESIAN_POINT ( 'NONE',  ( 17.18896242946999919, 60.50854855881860317, 20.47421955154796436 ) ) ;
#2455=ORIENTED_EDGE ( 'NONE', *, *, #2058, .T. ) ;
#2459=CARTESIAN_POINT ( 'NONE',  ( -39.18898618735786243, 44.43394377878069434, -18.33326528472845141 ) ) ;
#2464=DIRECTION ( 'NONE',  ( -1.000000000000000000, -0.000000000000000000, -0.000000000000000000 ) ) ;
#2468=CARTESIAN_POINT ( 'NONE',  ( -54.83316724383741558, 58.91257860089942255, 5.849939449132066649 ) ) ;
#2470=CARTESIAN_POINT ( 'NONE',  ( -15.09523335307150838, 60.00000000000000000, 4.640896189903090912E-12 ) ) ;
#2471=DIRECTION ( 'NONE',  ( 1.000000000000000000, 6.033820786006286457E-17, -0.000000000000000000 ) ) ;
#2473=AXIS2_PLACEMENT_3D ( 'NONE', #10582, #4368, #2511 ) ;
#2482=CARTESIAN_POINT ( 'NONE',  ( -20.09713505253791865, 55.00123338473885326, -0.01962842282139863267 ) ) ;
#2491=CARTESIAN_POINT ( 'NONE',  ( -19.21475903476782676, 67.52694740698208875, 16.89034408144044264 ) ) ;
#2492=CARTESIAN_POINT ( 'NONE',  ( -13.12707293678424136, 68.65161204859832367, -3.672914953887924661 ) ) ;
#2503=CARTESIAN_POINT ( 'NONE',  ( 22.64121015219242139, 59.33611995765907920, 2.510795356531756894 ) ) ;
#2504=CARTESIAN_POINT ( 'NONE',  ( -21.41713453776156939, 58.30068857233666790, 6.174842648405145518 ) ) ;
#2506=CARTESIAN_POINT ( 'NONE',  ( -6.596024235661785085, 64.91289939244650498, -18.55097902119702624 ) ) ;
#2511=DIRECTION ( 'NONE',  ( 0.000000000000000000, 1.000000000000000000, 0.000000000000000000 ) ) ;
#2517=CARTESIAN_POINT ( 'NONE',  ( -64.85481352702973368, 50.50649124814121649, 2.217451826950856297 ) ) ;
#2518=CARTESIAN_POINT ( 'NONE',  ( 11.81093755974026394, 42.10901286868706705, 16.77394813616862734 ) ) ;
#2522=CARTESIAN_POINT ( 'NONE',  ( -59.04091006144056308, 57.21723975501232218, 4.493613460639234169 ) ) ;
#2524=CARTESIAN_POINT ( 'NONE',  ( 10.18651522171044554, 52.78500897206648546, 4.494612666729983275 ) ) ;
#2531=CARTESIAN_POINT ( 'NONE',  ( -39.37536695926829111, 54.65609681119118335, -6.991488595795473771 ) ) ;
#2532=PLANE ( 'NONE',  #10533 ) ;
#2541=CARTESIAN_POINT ( 'NONE',  ( 1.092736580689907200, 55.00849556027373666, 0.02481302773033131764 ) ) ;
#2548=CARTESIAN_POINT ( 'NONE',  ( -54.78543919591579225, 71.88463165892282802, 12.52160998826382965 ) ) ;
#2549=CARTESIAN_POINT ( 'NONE',  ( -48.12707312818091765, 66.20688134294232441, -8.617576982512209938 ) ) ;
#2556=ORIENTED_EDGE ( 'NONE', *, *, #9539, .T. ) ;
#2559=CARTESIAN_POINT ( 'NONE',  ( 14.24053855247502121, 55.00473321740069821, 0.01576102579767488590 ) ) ;
#2561=CARTESIAN_POINT ( 'NONE',  ( -6.881425704338284710, 65.81090974167105401, -18.03733726640467694 ) ) ;
#2562=CARTESIAN_POINT ( 'NONE',  ( -19.88142569839470042, 67.52672413929985851, 16.89011978890229315 ) ) ;
#2565=AXIS2_PLACEMENT_3D ( 'NONE', #6837, #11414, #3892 ) ;
#2573=CARTESIAN_POINT ( 'NONE',  ( -62.51030605291772702, 43.28161195024001273, 17.55542603392786916 ) ) ;
#2582=CARTESIAN_POINT ( 'NONE',  ( 12.51356687061732664, 54.66830098263688598, 4.999997770403642683 ) ) ;
#2584=DIRECTION ( 'NONE',  ( 0.000000000000000000, 1.000000000000000000, 0.000000000000000000 ) ) ;
#2588=ORIENTED_EDGE ( 'NONE', *, *, #8050, .F. ) ;
#2590=CARTESIAN_POINT ( 'NONE',  ( 7.836421160393130414, 41.20749391036343212, 2.739689159572535448 ) ) ;
#2599=CARTESIAN_POINT ( 'NONE',  ( -57.99733838118905282, 54.99932032637487112, 0.003899505293572518017 ) ) ;
#2604=CARTESIAN_POINT ( 'NONE',  ( -19.92923235869172061, 55.82034979468773628, 4.934922690953704283 ) ) ;
#2607=CARTESIAN_POINT ( 'NONE',  ( -55.07084767368650091, 71.24562247638961310, 13.33442519937083404 ) ) ;
#2615=CARTESIAN_POINT ( 'NONE',  ( 21.86348472080128502, 58.97384788876435380, 3.051976829295043103 ) ) ;
#2616=CARTESIAN_POINT ( 'NONE',  ( -61.37538809735546863, 55.34397181478555439, 6.994694612480975238 ) ) ;
#2617=EDGE_LOOP ( 'NONE', ( #462, #2641, #2728, #1647 ) ) ;
#2618=CARTESIAN_POINT ( 'NONE',  ( -63.06671435217206323, 41.62111505249539078, 16.30162306856191989 ) ) ;
#2620=CARTESIAN_POINT ( 'NONE',  ( -40.60828084101493829, 48.86090744392433294, -20.20262880343927847 ) ) ;
#2626=DIRECTION ( 'NONE',  ( 1.000000000000000000, 6.033820786006286457E-17, 0.000000000000000000 ) ) ;
#2629=CARTESIAN_POINT ( 'NONE',  ( -44.39182476880109363, 68.38060868816502591, -16.29271878486493463 ) ) ;
#2633=CARTESIAN_POINT ( 'NONE',  ( -59.81854832799476185, 56.60795527072578182, 4.745860713526097285 ) ) ;
#2634=ORIENTED_EDGE ( 'NONE', *, *, #6057, .F. ) ;
#2641=ORIENTED_EDGE ( 'NONE', *, *, #3201, .T. ) ;
#2644=CARTESIAN_POINT ( 'NONE',  ( -7.287414961092598453, 58.76490461671014032, -3.306449428548710934 ) ) ;
#2645=CARTESIAN_POINT ( 'NONE',  ( -14.92871872213861018, 67.42576808392385601, 6.633445025436828679 ) ) ;
#2659=CARTESIAN_POINT ( 'NONE',  ( -25.90292780145558282, 54.98522453252181919, 0.01301329896340179364 ) ) ;
#2662=CARTESIAN_POINT ( 'NONE',  ( -11.96064323986153255, 59.99999999999997868, 0.3308892280880238457 ) ) ;
#2663=AXIS2_PLACEMENT_3D ( 'NONE', #5927, #7953, #9570 ) ;
#2667=CARTESIAN_POINT ( 'NONE',  ( -37.81096152632984797, 42.07775575353442576, -16.80518334814213333 ) ) ;
#2673=CARTESIAN_POINT ( 'NONE',  ( -26.94161418247137263, 38.68192823000178038, 13.40559829713685502 ) ) ;
#2678=CARTESIAN_POINT ( 'NONE',  ( -6.569594461653855078, 55.00124529901456327, -0.01228082968807806159 ) ) ;
#2679=VECTOR ( 'NONE', #482, 1000.000000000000000 ) ;
#2681=CARTESIAN_POINT ( 'NONE',  ( -65.17448922114576249, 36.67438677247554324, 10.54995967583099237 ) ) ;
#2682=CARTESIAN_POINT ( 'NONE',  ( 3.737309610555803463, 34.06887424008940712, -2.059134394038261817 ) ) ;
#2684=CYLINDRICAL_SURFACE ( 'NONE', #6703, 4.999999999999984013 ) ;
#2688=CARTESIAN_POINT ( 'NONE',  ( -40.24052535843971867, 55.00473963081345374, 0.01574568287803283437 ) ) ;
#2689=CARTESIAN_POINT ( 'NONE',  ( -62.51716279675893873, 51.69589315519270656, 3.766953055518623472 ) ) ;
#2692=DIRECTION ( 'NONE',  ( 0.000000000000000000, 1.000000000000000000, 0.000000000000000000 ) ) ;
#2695=CARTESIAN_POINT ( 'NONE',  ( -69.53699434246021838, 50.16068223471152265, 1.299115590555422139 ) ) ;
#2699=CARTESIAN_POINT ( 'NONE',  ( 47.00000000000000000, 51.46446609406726935, -3.535533905932743526 ) ) ;
#2707=ORIENTED_EDGE ( 'NONE', *, *, #11755, .F. ) ;
#2708=CARTESIAN_POINT ( 'NONE',  ( -4.954815148401325864, 57.21385113419372459, -4.495241971010075943 ) ) ;
#2709=CARTESIAN_POINT ( 'NONE',  ( 1.206260390864687171, 46.37779328219373554, -11.21151207404757066 ) ) ;
#2714=AXIS2_PLACEMENT_3D ( 'NONE', #875, #819, #2692 ) ;
#2720=CARTESIAN_POINT ( 'NONE',  ( -33.09269368653934151, 54.97643580162243637, -0.01155639149150148627 ) ) ;
#2725=EDGE_CURVE ( 'NONE', #658, #7013, #7610, .T. ) ;
#2726=B_SPLINE_CURVE_WITH_KNOTS ( 'NONE', 3,
 ( #10652, #3416, #6971, #9707 ),
 .UNSPECIFIED., .F., .F.,
 ( 4, 4 ),
 ( 0.0003222502065252045981, 0.003846531889534238625 ),
 .UNSPECIFIED. ) ;
#2727=DIRECTION ( 'NONE',  ( 0.000000000000000000, 1.000000000000000000, 0.000000000000000000 ) ) ;
#2728=ORIENTED_EDGE ( 'NONE', *, *, #6109, .F. ) ;
#2731=CARTESIAN_POINT ( 'NONE',  ( -9.969360172258976860, 70.58303384883494402, -14.12411716821732277 ) ) ;
#2736=CARTESIAN_POINT ( 'NONE',  ( -24.81096152833125856, 44.41791055217656492, 18.37268719335390443 ) ) ;
#2737=EDGE_LOOP ( 'NONE', ( #1207, #1028, #1467, #536 ) ) ;
#2739=CARTESIAN_POINT ( 'NONE',  ( -10.95223875328497343, 55.00428177097578697, -0.003223779858058093296 ) ) ;
#2741=CARTESIAN_POINT ( 'NONE',  ( -18.54809237114100284, 67.52717067466427636, 16.89056837398185351 ) ) ;
#2742=CARTESIAN_POINT ( 'NONE',  ( -33.30269350532120143, 33.99387206627966407, -1.031609878214063025 ) ) ;
#2744=( LENGTH_UNIT ( ) NAMED_UNIT ( * ) SI_UNIT ( .MILLI., .METRE. ) );
#2749=CARTESIAN_POINT ( 'NONE',  ( -35.16317177855322029, 54.99748849700297626, -0.0002045196618292968900 ) ) ;
#2750=CARTESIAN_POINT ( 'NONE',  ( -45.01221456438528890, 58.97241515813631452, -3.054071859287629032 ) ) ;
#2756=CARTESIAN_POINT ( 'NONE',  ( -66.47562283042974229, 38.19906477560226676, 12.92409071120044040 ) ) ;
#2759=VERTEX_POINT ( 'NONE', #4071 ) ;
#2763=CARTESIAN_POINT ( 'NONE',  ( -17.25615151965529037, 63.89925965980745559, 10.84111801642336026 ) ) ;
#2773=CARTESIAN_POINT ( 'NONE',  ( -39.04772848043890576, 54.99975663035424134, 0.008780986960116223677 ) ) ;
#2781=CARTESIAN_POINT ( 'NONE',  ( -4.188986194789085182, 52.25407379690145859, -20.98118322582191908 ) ) ;
#2786=CARTESIAN_POINT ( 'NONE',  ( -40.33720992201957500, 55.00042869323097960, -21.02810349118288258 ) ) ;
#2790=CARTESIAN_POINT ( 'NONE',  ( 19.14436220527237253, 71.77763100192429135, 12.89423484158165500 ) ) ;
#2793=CARTESIAN_POINT ( 'NONE',  ( -27.60828084806726324, 38.68279673837142241, 13.40472996373423520 ) ) ;
#2794=CARTESIAN_POINT ( 'NONE',  ( -1.855729112296511385, 44.43418165317581980, -18.33336562707187412 ) ) ;
#2800=EDGE_CURVE ( 'NONE', #11420, #1911, #7728, .T. ) ;
#2803=CARTESIAN_POINT ( 'NONE',  ( -57.61887970616808730, 55.00322141028932776, 0.004312430475834024002 ) ) ;
#2804=CARTESIAN_POINT ( 'NONE',  ( -39.18048067635331932, 54.66929070781851152, -5.000014872209115779 ) ) ;
#2805=CARTESIAN_POINT ( 'NONE',  ( 52.99999999999999289, 55.00000000000000000, 3.000000000000002665 ) ) ;
#2807=ORIENTED_EDGE ( 'NONE', *, *, #10917, .T. ) ;
#2808=CARTESIAN_POINT ( 'NONE',  ( 18.81101721030213625, 65.56418867429738384, 18.32872549916029925 ) ) ;
#2809=CARTESIAN_POINT ( 'NONE',  ( -32.98217015207742264, 50.00000000000001421, 0.6598160721750869762 ) ) ;
#2819=CARTESIAN_POINT ( 'NONE',  ( -8.503152583179597102, 66.69685394566769787, -7.822304719850006194 ) ) ;
#2828=CARTESIAN_POINT ( 'NONE',  ( -58.57658864237733809, 54.99919238257378851, 0.009360382064782520051 ) ) ;
#2829=PRODUCT_CONTEXT ( 'NONE', #7011, 'mechanical' ) ;
#2830=AXIS2_PLACEMENT_3D ( 'NONE', #3481, #8929, #11840 ) ;
#2832=CARTESIAN_POINT ( 'NONE',  ( 62.44550000000000267, 55.00000000000000000, 0.000000000000000000 ) ) ;
#2834=CARTESIAN_POINT ( 'NONE',  ( 9.813847082697366275, 50.50592320711870542, 2.216018654255096809 ) ) ;
#2837=CARTESIAN_POINT ( 'NONE',  ( 12.14423903554155793, 49.50741477678717928, 20.43476828740966766 ) ) ;
#2842=CARTESIAN_POINT ( 'NONE',  ( -41.78535879711923684, 60.10680040617825881, -20.39053309953287751 ) ) ;
#2845=PLANE ( 'NONE',  #6829 ) ;
#2847=CARTESIAN_POINT ( 'NONE',  ( -4.983946421173099495, 54.34173040065561366, -4.967129911086819227 ) ) ;
#2848=CARTESIAN_POINT ( 'NONE',  ( -5.608280846031337141, 57.05942937149918492, -21.01412426850803783 ) ) ;
#2850=CARTESIAN_POINT ( 'NONE',  ( -53.26270066237940171, 73.55098385638794412, 9.912901411881726688 ) ) ;
#2852=CARTESIAN_POINT ( 'NONE',  ( -46.39182477221876866, 68.38321102182860045, -16.29532114285349920 ) ) ;
#2860=CARTESIAN_POINT ( 'NONE',  ( -58.49661103985690858, 55.00163715208778825, 0.001795710856485419104 ) ) ;
#2861=CARTESIAN_POINT ( 'NONE',  ( -35.28845012686586102, 51.69504605834636379, -3.766257009993432270 ) ) ;
#2867=CARTESIAN_POINT ( 'NONE',  ( 3.957967453204893626, 48.00580430340492200, 0.3439981469349869259 ) ) ;
#2869=CARTESIAN_POINT ( 'NONE',  ( 6.329456780446692576, 33.97189653527247089, -0.0004287163746460355418 ) ) ;
#2883=CARTESIAN_POINT ( 'NONE',  ( -46.20623825043654875, 67.21094750618843250, -7.039791742250042894 ) ) ;
#2887=CARTESIAN_POINT ( 'NONE',  ( 36.99999999999999289, 59.99999999999998579, 0.000000000000000000 ) ) ;
#2892=CARTESIAN_POINT ( 'NONE',  ( -33.76207074264209496, 50.00000000000002842, -7.785926851161516095E-15 ) ) ;
#2894=CARTESIAN_POINT ( 'NONE',  ( 8.166442932151195322, 48.10666307911134254, 1.369977444835037028 ) ) ;
#2903=CARTESIAN_POINT ( 'NONE',  ( -20.45202553191040806, 65.80759480864719535, 18.03021102644938267 ) ) ;
#2908=CARTESIAN_POINT ( 'NONE',  ( -19.32947785509334082, 63.04547287423799418, 19.42212676744230393 ) ) ;
#2909=FILL_AREA_STYLE_COLOUR ( '', #1043 ) ;
#2911=CARTESIAN_POINT ( 'NONE',  ( -59.59556320886013481, 52.94111634316250559, 20.93276532467568174 ) ) ;
#2914=CARTESIAN_POINT ( 'NONE',  ( -0.7106829068669191507, 51.23386462371114902, -3.305037806040365123 ) ) ;
#2917=CARTESIAN_POINT ( 'NONE',  ( -20.30269393938554501, 62.08599396958958039, 19.80292882502584817 ) ) ;
#2918=CARTESIAN_POINT ( 'NONE',  ( -62.73530513678402087, 48.89572068339310107, 20.11073150603193938 ) ) ;
#2919=LINE ( 'NONE', #4109, #5655 ) ;
#2920=CARTESIAN_POINT ( 'NONE',  ( 24.99999999999999645, 76.00000000000000000, 0.000000000000000000 ) ) ;
#2925=CARTESIAN_POINT ( 'NONE',  ( -29.90292779502757270, 54.99043558275273114, 0.007803298580286864745 ) ) ;
#2926=CARTESIAN_POINT ( 'NONE',  ( -38.79059579792235013, 54.34011855466147978, -4.966942020943686309 ) ) ;
#2929=CARTESIAN_POINT ( 'NONE',  ( 5.417510076880946990, 48.25790868973780334, 2.048730295261496082 ) ) ;
#2943=CARTESIAN_POINT ( 'NONE',  ( -64.12603728547384208, 43.79068664598788274, 8.623361052036228713 ) ) ;
#2952=CARTESIAN_POINT ( 'NONE',  ( -36.48177824941181058, 50.50603341324405449, -2.216217228574558273 ) ) ;
#2955=CARTESIAN_POINT ( 'NONE',  ( 22.55679944818120575, 61.13996205570565934, 3.535017745053270044 ) ) ;
#2957=DIRECTION ( 'NONE',  ( -1.000000000000000000, -0.000000000000000000, -0.000000000000000000 ) ) ;
#2959=DIRECTION ( 'NONE',  ( 1.000000000000000000, 6.033820786006286457E-17, -0.000000000000000000 ) ) ;
#2962=CARTESIAN_POINT ( 'NONE',  ( -10.83980928483403794, 72.54296691076741865, -11.73126556815853760 ) ) ;
#2965=CARTESIAN_POINT ( 'NONE',  ( -65.17448922114576249, 36.67438677247554324, 10.54995967583099237 ) ) ;
#2968=DIRECTION ( 'NONE',  ( 0.000000000000000000, 1.000000000000000000, 0.000000000000000000 ) ) ;
#2969=FACE_OUTER_BOUND ( 'NONE', #2000, .T. ) ;
#2970=CARTESIAN_POINT ( 'NONE',  ( 16.81101720596863203, 65.56606704192360269, 18.33326034385300574 ) ) ;
#2973=CARTESIAN_POINT ( 'NONE',  ( -19.99614452984508262, 63.04554348432252198, 19.42230297928623628 ) ) ;
#2974=CARTESIAN_POINT ( 'NONE',  ( 4.296995438882074581, 41.00607614374722942, 0.6876389650848340196 ) ) ;
#2976=DIRECTION ( 'NONE',  ( -6.033820786006286457E-17, 1.000000000000000000, 0.000000000000000000 ) ) ;
#2987=CARTESIAN_POINT ( 'NONE',  ( 21.55487747176179170, 62.01724152347335917, 0.9185355870624294372 ) ) ;
#2990=DIRECTION ( 'NONE',  ( 0.000000000000000000, 0.000000000000000000, -1.000000000000000000 ) ) ;
#2991=DIRECTION ( 'NONE',  ( -1.000000000000000000, -6.033820786006286457E-17, -0.000000000000000000 ) ) ;
#3000=CARTESIAN_POINT ( 'NONE',  ( -38.26205205313807056, 50.90420908871833205, -13.47689883053113213 ) ) ;
#3006=AXIS2_PLACEMENT_3D ( 'NONE', #94, #2079, #2017 ) ;
#3010=ADVANCED_FACE ( 'NONE', ( #10697 ), #4999, .T. ) ;
#3011=CARTESIAN_POINT ( 'NONE',  ( -22.55675198223577027, 53.17748975554098934, 6.794389702512826368 ) ) ;
#3021=CARTESIAN_POINT ( 'NONE',  ( -27.52231952827322559, 42.10572610250680015, 16.77759997522909785 ) ) ;
#3031=CARTESIAN_POINT ( 'NONE',  ( 2.595920079249742329, 34.88763922991881827, -6.102757042485290384 ) ) ;
#3033=CARTESIAN_POINT ( 'NONE',  ( -6.670543235071888510, 63.04736075021470754, -19.42691569015581976 ) ) ;
#3034=CARTESIAN_POINT ( 'NONE',  ( 2.256059437406555457, 41.59371342422682716, -4.067545439913939020 ) ) ;
#3046=CARTESIAN_POINT ( 'NONE',  ( -63.07624402531011754, 50.93185762523746973, 13.40497886217843160 ) ) ;
#3047=VERTEX_POINT ( 'NONE', #7602 ) ;
#3048=CARTESIAN_POINT ( 'NONE',  ( -6.785358873008338954, 67.52118754941005818, -16.88410835930674381 ) ) ;
#3050=B_SPLINE_CURVE_WITH_KNOTS ( 'NONE', 3,
 ( #9374, #8542, #11038, #5674, #2790, #8487, #2970, #325, #1044, #11221, #3990, #7650, #5738, #4709, #7479, #6700, #4768, #142, #3808, #8301, #1166, #9315, #3031, #10331, #6454, #1882, #9196, #987, #11100, #82, #3744, #2848, #6517, #6580, #2003, #10615, #11341, #8609, #387, #4285, #4104, #11283, #3096, #3149, #2425, #4953, #6936, #6762, #4163, #1352, #10389, #3265, #4055, #2365, #7711, #5132, #2245, #8666, #6037, #7762, #2185, #6817, #5190, #7887, #5983, #2306, #8842, #5018, #1526, #8718, #10442, #446, #5855, #9558, #11393, #1469, #5914, #3206, #6875, #561, #501, #621, #1412, #9672, #10502, #6094, #9496, #9617, #5074, #1286, #7823, #11456, #8780, #10564, #4228, #11518, #3324, #6992, #9726, #677, #5365, #4350, #9017, #5250, #6274, #11577, #7942, #9789, #4467, #6153, #6332, #8897, #5422, #9961, #9072, #848, #10916, #3379, #7232, #4519, #7170, #793, #1809, #10739 ),
 .UNSPECIFIED., .F., .F.,
 ( 4, 2, 2, 2, 2, 2, 2, 2, 2, 2, 2, 2, 2, 2, 2, 2, 2, 2, 2, 2, 2, 2, 2, 2, 2, 2, 2, 2, 2, 2, 2, 2, 2, 2, 2, 2, 2, 2, 2, 2, 2, 2, 2, 2, 2, 2, 2, 2, 2, 2, 2, 2, 2, 2, 2, 2, 2, 2, 2, 2, 2, 4 ),
 ( 0.000000000000000000, 0.02499977550252127645, 0.04999988577693819519, 0.07499999605135511394, 0.09999999831535408279, 0.1250000005793530378, 0.1500000028441162425, 0.1750000051088794195, 0.1937500039558066045, 0.2031250033792701970, 0.2125000028027338173, 0.2218750022261974375, 0.2312500016496610300, 0.2500000004965882150, 0.2750000027613288545, 0.3000000050260694384, 0.3187500038730080032, 0.3281250032964772578, 0.3375000027199465125, 0.3468750021434158226, 0.3562500015668850772, 0.3750000004138236420, 0.4000000026785641705, 0.4250000049433046989, 0.4437500037902432082, 0.4531250032137125183, 0.4625000026371817730, 0.4718750020606510276, 0.4812500014841203377, 0.5000000003310588470, 0.5250000025957997085, 0.5500000048605405700, 0.5687500037074788573, 0.5781250031309480564, 0.5875000025544172555, 0.5968750019778864546, 0.6062500014013556537, 0.6250000002482940520, 0.6500000025128280789, 0.6750000047773621059, 0.6937500036244039769, 0.7031250030479249125, 0.7125000024714458480, 0.7218750018949667835, 0.7312500013184877190, 0.7500000001655295900, 0.7750000023794885173, 0.8000000045934475557, 0.8187500034657768655, 0.8281250029019414649, 0.8375000023381060643, 0.8468750017742707747, 0.8562500012104353742, 0.8750000000827646840, 0.8937502654913498379, 0.9031253981956424148, 0.9125005308999349918, 0.9218756636042275687, 0.9312507963085201457, 0.9500010617171052996, 0.9750005308585526498, 1.000000000000000000 ),
 .UNSPECIFIED. ) ;
#3051=DIRECTION ( 'NONE',  ( 0.000000000000000000, 0.000000000000000000, 1.000000000000000000 ) ) ;
#3061=CARTESIAN_POINT ( 'NONE',  ( -28.92281818629570722, 41.57851372300513049, 4.073127600961401029 ) ) ;
#3066=CIRCLE ( 'NONE', #10119, 9.999999999999987566 ) ;
#3070=CARTESIAN_POINT ( 'NONE',  ( -49.71141041926628645, 59.49513311707226393, -2.214139657851166287 ) ) ;
#3073=CARTESIAN_POINT ( 'NONE',  ( -1.556678960741344708, 54.08359337848497006, -6.974639707943993017 ) ) ;
#3081=CARTESIAN_POINT ( 'NONE',  ( -43.78535878948660098, 60.10716095388539060, -20.39140800440753054 ) ) ;
#3086=CARTESIAN_POINT ( 'NONE',  ( -61.63584152524990145, 46.00569487729882212, 19.01260273971552905 ) ) ;
#3093=CARTESIAN_POINT ( 'NONE',  ( -1.482474291011559364, 51.69668081413308158, -3.767642887559051079 ) ) ;
#3095=EDGE_CURVE ( 'NONE', #1776, #5647, #9569, .T. ) ;
#3096=CARTESIAN_POINT ( 'NONE',  ( -11.39182375260447166, 73.60042400440836730, -9.933379572949093017 ) ) ;
#3097=ORIENTED_EDGE ( 'NONE', *, *, #291, .T. ) ;
#3098=CARTESIAN_POINT ( 'NONE',  ( 4.996123431639940549, 33.97227858069939543, -0.0004331113196134536714 ) ) ;
#3100=CARTESIAN_POINT ( 'NONE',  ( -56.63607177307330431, 69.12418599258134577, 15.58301102096070245 ) ) ;
#3110=CARTESIAN_POINT ( 'NONE',  ( 12.22341952602966764, 54.08367749976515171, 7.017190178460947614 ) ) ;
#3112=CARTESIAN_POINT ( 'NONE',  ( -37.18898618307433424, 44.43582214169357769, -18.32873044267784479 ) ) ;
#3122=CARTESIAN_POINT ( 'NONE',  ( -60.12103580250087731, 51.59597441208588720, 13.59059695706972626 ) ) ;
#3132=CARTESIAN_POINT ( 'NONE',  ( -16.91627854707998679, 59.45272466182848348, 5.424304687769180511 ) ) ;
#3134=DIRECTION ( 'NONE',  ( 0.000000000000000000, 0.000000000000000000, 1.000000000000000000 ) ) ;
#3136=DIRECTION ( 'NONE',  ( 0.000000000000000000, 1.000000000000000000, 0.000000000000000000 ) ) ;
#3139=CARTESIAN_POINT ( 'NONE',  ( -23.05849041873830885, 57.05917197429855037, 20.98589082339331569 ) ) ;
#3143=CARTESIAN_POINT ( 'NONE',  ( -60.73530621856283318, 48.89645762657089278, 20.10868697360108115 ) ) ;
#3149=CARTESIAN_POINT ( 'NONE',  ( -12.81092923270300865, 75.46953867936616689, -5.507006106411301616 ) ) ;
#3151=CARTESIAN_POINT ( 'NONE',  ( -69.00771387827577996, 33.99486225849476995, 0.006699851613120169809 ) ) ;
#3152=CARTESIAN_POINT ( 'NONE',  ( -34.50315233865081410, 41.19915729885462952, -2.739730459386737316 ) ) ;
#3158=CARTESIAN_POINT ( 'NONE',  ( -61.99733827119050744, 54.99927236536940711, 0.002460332904419732219 ) ) ;
#3163=CARTESIAN_POINT ( 'NONE',  ( -14.22341865602713007, 61.98282206426377883, -0.9163204132140592151 ) ) ;
#3165=CARTESIAN_POINT ( 'NONE',  ( -50.82691677660828589, 75.68920158268997511, 4.121780573430135597 ) ) ;
#3173=ORIENTED_EDGE ( 'NONE', *, *, #2725, .F. ) ;
#3177=CARTESIAN_POINT ( 'NONE',  ( -25.52231952398968673, 42.10919693116569817, 16.77412918608628090 ) ) ;
#3179=CARTESIAN_POINT ( 'NONE',  ( 34.00000000000000000, 59.99999999999998579, 0.000000000000000000 ) ) ;
#3188=CARTESIAN_POINT ( 'NONE',  ( -48.22334500059429274, 61.97465389400121438, -0.9164071902225618960 ) ) ;
#3193=CIRCLE ( 'NONE', #3006, 4.999999999999997335 ) ;
#3196=EDGE_LOOP ( 'NONE', ( #7308, #9981 ) ) ;
#3201=EDGE_CURVE ( 'NONE', #4223, #10886, #6281, .T. ) ;
#3204=B_SPLINE_CURVE_WITH_KNOTS ( 'NONE', 3,
 ( #5615, #2127, #3989, #4889, #5737, #1042, #3806, #4708, #11281, #5800, #2914, #3093, #9434, #8360, #4767, #6579, #10209, #2847, #10083, #2002, #1222, #7649, #1880, #986, #1164, #9195, #4834, #8486, #7590, #4647, #8422, #8300, #80, #3743, #11559, #10441, #9772, #2470 ),
 .UNSPECIFIED., .F., .F.,
 ( 4, 2, 2, 2, 2, 2, 2, 2, 2, 2, 2, 2, 2, 2, 2, 2, 2, 2, 4 ),
 ( 0.02428446548970041724, 0.02580228911461803637, 0.02732011273953565550, 0.02807902455199446506, 0.02883793636445327463, 0.03035575998937089376, 0.03187358361428851289, 0.03339140723920613202, 0.03490923086412375115, 0.03642705448904137028, 0.03794487811395898247, 0.03946270173887660854, 0.04022161355133541810, 0.04098052536379422767, 0.04249834898871186067, 0.04401617261362950062, 0.04553399623854713363, 0.04705181986346476664, 0.04856964348838239964 ),
 .UNSPECIFIED. ) ;
#3206=CARTESIAN_POINT ( 'NONE',  ( -38.47762819156672265, 42.07891330237754346, -16.80402559754432801 ) ) ;
#3209=CARTESIAN_POINT ( 'NONE',  ( -18.03064345808105173, 70.57358235614606201, 14.11515935890559881 ) ) ;
#3210=CARTESIAN_POINT ( 'NONE',  ( -43.25615049311128502, 56.37302494055165170, -13.95606205737922423 ) ) ;
#3213=CARTESIAN_POINT ( 'NONE',  ( -18.20729755437997710, 59.33894261634819145, 2.506317759643504228 ) ) ;
#3218=CIRCLE ( 'NONE', #9909, 9.999999999999987566 ) ;
#3220=CARTESIAN_POINT ( 'NONE',  ( -29.58248992310308978, 49.55513497353873476, 4.472866631367526935 ) ) ;
#3222=CARTESIAN_POINT ( 'NONE',  ( -51.69727455458300369, 74.78870212167194609, 7.080596778485133136 ) ) ;
#3223=CARTESIAN_POINT ( 'NONE',  ( 21.47754340280339136, 75.43473409906381733, 5.492671141289128478 ) ) ;
#3224=EDGE_CURVE ( 'NONE', #678, #1342, #682, .T. ) ;
#3233=CARTESIAN_POINT ( 'NONE',  ( -15.82693394478133797, 72.53700911420227726, 11.72543866452437733 ) ) ;
#3243=CIRCLE ( 'NONE', #4970, 4.999999999999997335 ) ;
#3245=CARTESIAN_POINT ( 'NONE',  ( -46.20572079224533724, 57.50577717681836276, -4.339287318856722919 ) ) ;
#3247=CARTESIAN_POINT ( 'NONE',  ( -38.50022373450124036, 53.63002255421522335, -6.893336926830083478 ) ) ;
#3249=CARTESIAN_POINT ( 'NONE',  ( 36.99999999999999289, 50.00000000000001421, 6.123233995736750505E-16 ) ) ;
#3258=CARTESIAN_POINT ( 'NONE',  ( 20.57387831814119750, 55.01735003982987138, 0.01969578267603667651 ) ) ;
#3265=CARTESIAN_POINT ( 'NONE',  ( -19.59602372284622618, 68.34451306940553650, 16.25656885606184332 ) ) ;
#3266=VERTEX_POINT ( 'NONE', #9912 ) ;
#3267=CARTESIAN_POINT ( 'NONE',  ( 3.547974465258201704, 34.60888357062293608, -5.107040723657290116 ) ) ;
#3268=CARTESIAN_POINT ( 'NONE',  ( -7.668535110823559542, 60.36516981310766283, -12.95174721521620853 ) ) ;
#3270=CARTESIAN_POINT ( 'NONE',  ( -25.21223637683726793, 54.34188354068985660, 4.967192001377610744 ) ) ;
#3277=LINE ( 'NONE', #5929, #5493 ) ;
#3278=CIRCLE ( 'NONE', #11311, 4.999999999999997335 ) ;
#3279=CARTESIAN_POINT ( 'NONE',  ( -54.37536708495734672, 61.59341897336967264, 2.358744290958179057 ) ) ;
#3281=CARTESIAN_POINT ( 'NONE',  ( -18.73741402030934111, 64.90551912913463184, 18.53518525054827393 ) ) ;
#3283=CARTESIAN_POINT ( 'NONE',  ( 6.058385820703728442, 34.79737119409461599, 6.139092558150637480 ) ) ;
#3294=CARTESIAN_POINT ( 'NONE',  ( -17.59602449223222109, 68.34579465778965357, 16.25793134507749826 ) ) ;
#3308=CARTESIAN_POINT ( 'NONE',  ( -62.41739093814645400, 50.54543071709656488, 5.426587404619046318 ) ) ;
#3310=EDGE_CURVE ( 'NONE', #1626, #5647, #1364, .T. ) ;
#3320=CARTESIAN_POINT ( 'NONE',  ( -5.204882849839850500, 55.00196753710881836, -0.004080773591198232075 ) ) ;
#3324=CARTESIAN_POINT ( 'NONE',  ( -52.82691659388441252, 75.69008924411679118, 4.122156975067814422 ) ) ;
#3326=CARTESIAN_POINT ( 'NONE',  ( -18.92935731264207888, 68.34494026553466028, 16.25702301906597569 ) ) ;
#3327=CARTESIAN_POINT ( 'NONE',  ( -9.410607229192429202, 63.88828574158252138, -10.82921152398832021 ) ) ;
#3335=CARTESIAN_POINT ( 'NONE',  ( -25.89008532269601659, 53.17435935992097029, 6.801947025163535443 ) ) ;
#3337=CARTESIAN_POINT ( 'NONE',  ( -46.52239103091250172, 73.32882989972571863, -10.56393531560676102 ) ) ;
#3346=CARTESIAN_POINT ( 'NONE',  ( -5.929357825456832209, 64.91315550346766372, -18.55154749960842153 ) ) ;
#3349=CARTESIAN_POINT ( 'NONE',  ( -64.47634457867742697, 52.78883415961983872, 4.496407241981684955 ) ) ;
#3352=CARTESIAN_POINT ( 'NONE',  ( -34.17314261869798742, 34.29999169977881479, -4.109493429249395646 ) ) ;
#3356=DIRECTION ( 'NONE',  ( 1.000000000000000000, 6.033820786006286457E-17, -0.000000000000000000 ) ) ;
#3357=VERTEX_POINT ( 'NONE', #3921 ) ;
#3360=CARTESIAN_POINT ( 'NONE',  ( -27.99986027349028817, 48.52216085064172546, 2.682930977694029551 ) ) ;
#3361=DIRECTION ( 'NONE',  ( -6.033820786006286457E-17, 1.000000000000000000, 0.000000000000000000 ) ) ;
#3373=CARTESIAN_POINT ( 'NONE',  ( 17.42607031566902975, 55.00164666455483342, -0.02617539568509523462 ) ) ;
#3377=CARTESIAN_POINT ( 'NONE',  ( -27.71226046275158694, 50.44280945467068022, 2.063697696152629213 ) ) ;
#3379=CARTESIAN_POINT ( 'NONE',  ( -64.51030549024622474, 43.28227691760346119, 17.55408017169854418 ) ) ;
#3381=CARTESIAN_POINT ( 'NONE',  ( -35.47759590132267249, 36.63029660218667516, -10.58073486798289409 ) ) ;
#3382=CARTESIAN_POINT ( 'NONE',  ( -32.74394056260254615, 41.05762397541256803, 1.372441782585282155 ) ) ;
#3388=CARTESIAN_POINT ( 'NONE',  ( 23.47754340821147068, 75.43020022661498558, 5.490793176664390707 ) ) ;
#3393=CARTESIAN_POINT ( 'NONE',  ( 13.70862763294794640, 52.78289059355582680, 4.493706804602685345 ) ) ;
#3394=CARTESIAN_POINT ( 'NONE',  ( -10.33346892558120800, 59.95411981434817505, -4.954567573143832782 ) ) ;
#3397=CARTESIAN_POINT ( 'NONE',  ( -2.855652858599348143, 52.25407377826859801, -20.97791091579992440 ) ) ;
#3400=EDGE_CURVE ( 'NONE', #567, #7749, #8660, .T. ) ;
#3406=CARTESIAN_POINT ( 'NONE',  ( -66.01541562873828184, 50.16044088320995087, 1.297932126172365752 ) ) ;
#3408=CARTESIAN_POINT ( 'NONE',  ( -6.785358873008338954, 67.52118754941005818, -16.88410835930674381 ) ) ;
#3411=CARTESIAN_POINT ( 'NONE',  ( -62.14557957614105277, 54.67521725067852856, 5.000265375653349942 ) ) ;
#3413=CARTESIAN_POINT ( 'NONE',  ( -54.00383531698385298, 74.42670172875287449, 8.047314657126378279 ) ) ;
#3416=CARTESIAN_POINT ( 'NONE',  ( -69.91923606153405046, 50.00000003590698583, -0.0006041109642164819819 ) ) ;
#3422=CARTESIAN_POINT ( 'NONE',  ( 23.79370066466821498, 68.61228347134048988, 3.656683429161660115 ) ) ;
#3428=AXIS2_PLACEMENT_3D ( 'NONE', #8541, #9314, #324 ) ;
#3435=CARTESIAN_POINT ( 'NONE',  ( 13.57397298349323123, 54.98844360358936001, 0.02356420128931584895 ) ) ;
#3438=VECTOR ( 'NONE', #539, 1000.000000000000000 ) ;
#3441=CARTESIAN_POINT ( 'NONE',  ( -25.18353888624136516, 51.69772872632766791, 3.768611304527443640 ) ) ;
#3444=CARTESIAN_POINT ( 'NONE',  ( -33.50647601322769731, 34.29967001110087210, -4.109490822278082156 ) ) ;
#3445=CARTESIAN_POINT ( 'NONE',  ( -51.20617496588531026, 68.98201131862417412, -1.831174229402957820 ) ) ;
#3447=ADVANCED_FACE ( 'NONE', ( #6987 ), #11382, .T. ) ;
#3453=CARTESIAN_POINT ( 'NONE',  ( 24.99999999999999645, 76.00000000000000000, 0.000000000000000000 ) ) ;
#3457=ADVANCED_FACE ( 'NONE', ( #11096 ), #2845, .T. ) ;
#3460=CARTESIAN_POINT ( 'NONE',  ( 16.03565078256021437, 54.66604247513213011, 4.999734568126702250 ) ) ;
#3461=CARTESIAN_POINT ( 'NONE',  ( 2.756929297555888780, 54.99406534603833308, -0.0008060267085826582035 ) ) ;
#3464=CARTESIAN_POINT ( 'NONE',  ( -5.697310340841898579, 62.08076523182673867, -19.78924413987668629 ) ) ;
#3466=CARTESIAN_POINT ( 'NONE',  ( -12.81092923270300865, 75.46953867936616689, -5.507006106411301616 ) ) ;
#3475=CARTESIAN_POINT ( 'NONE',  ( -58.69833756168564065, 56.03204939003842355, 20.99267139547387373 ) ) ;
#3476=VECTOR ( 'NONE', #9982, 1000.000000000000000 ) ;
#3481=CARTESIAN_POINT ( 'NONE',  ( 53.00000000000000000, 51.46446609406726935, 3.535533905932731091 ) ) ;
#3486=PLANE ( 'NONE',  #200 ) ;
#3489=CARTESIAN_POINT ( 'NONE',  ( 5.211360173331719636, 41.40800266049619438, -3.403751673813347089 ) ) ;
#3498=CARTESIAN_POINT ( 'NONE',  ( 15.90727646477327717, 54.99834087400687821, 0.02619391509296356210 ) ) ;
#3505=CARTESIAN_POINT ( 'NONE',  ( -52.16024998812459756, 75.68979335697233068, 4.122031507855797194 ) ) ;
#3510=ORIENTED_EDGE ( 'NONE', *, *, #151, .T. ) ;
#3512=CARTESIAN_POINT ( 'NONE',  ( 24.20135950461900265, 59.84025108871626486, 1.295421926073733410 ) ) ;
#3513=CARTESIAN_POINT ( 'NONE',  ( -59.91576240004388154, 57.04875898427261660, 6.741986199795334755 ) ) ;
#3515=CARTESIAN_POINT ( 'NONE',  ( 16.52229576424834079, 60.50792211291388867, 20.47270680267081389 ) ) ;
#3516=CARTESIAN_POINT ( 'NONE',  ( -36.14426256656389569, 36.63180902967581432, -10.58010824564746599 ) ) ;
#3525=CARTESIAN_POINT ( 'NONE',  ( -42.96936073659074395, 63.99245613053683712, -19.01383356661934343 ) ) ;
#3533=CARTESIAN_POINT ( 'NONE',  ( 20.29449446700749959, 59.74572742522828861, 1.608070810192847810 ) ) ;
#3538=ORIENTED_EDGE ( 'NONE', *, *, #1824, .T. ) ;
#3539=CARTESIAN_POINT ( 'NONE',  ( 2.046876773580067255, 51.69375302741990907, -3.765136267534306747 ) ) ;
#3540=CARTESIAN_POINT ( 'NONE',  ( 6.963661241466286178, 41.00824184081660917, 0.6875629968608463205 ) ) ;
#3548=ORIENTED_EDGE ( 'NONE', *, *, #4766, .F. ) ;
#3555=CARTESIAN_POINT ( 'NONE',  ( -27.66451880046085776, 54.99704050659160259, 0.001041102682434957849 ) ) ;
#3559=CARTESIAN_POINT ( 'NONE',  ( -13.51214745100933357, 59.74687554544813395, 1.604952281176790230 ) ) ;
#3562=CARTESIAN_POINT ( 'NONE',  ( -30.00387656835589212, 35.57275282082603240, 8.046560464864068507 ) ) ;
#3565=ORIENTED_EDGE ( 'NONE', *, *, #10114, .F. ) ;
#3566=PRODUCT_DEFINITION_SHAPE ( 'NONE', 'NONE',  #4545 ) ;
#3569=CARTESIAN_POINT ( 'NONE',  ( -20.50647613538409075, 59.12524989819403487, 20.69783765389080799 ) ) ;
#3573=CARTESIAN_POINT ( 'NONE',  ( 21.24062560320400550, 55.01638079892301647, 0.001655951099807092403 ) ) ;
#3575=CARTESIAN_POINT ( 'NONE',  ( -59.59556320886013481, 52.94111634316250559, 20.93276532467568174 ) ) ;
#3577=CARTESIAN_POINT ( 'NONE',  ( -21.63602683877659771, 62.08561388645346568, 19.80191166437241179 ) ) ;
#3582=ORIENTED_EDGE ( 'NONE', *, *, #10114, .T. ) ;
#3585=CARTESIAN_POINT ( 'NONE',  ( -43.85119715763887882, 58.30290808985935769, -3.768050382088650618 ) ) ;
#3588=CARTESIAN_POINT ( 'NONE',  ( 7.095683716263478047, 50.00000000000005684, 2.757939276259992832E-15 ) ) ;
#3590=CARTESIAN_POINT ( 'NONE',  ( -65.64956124500029944, 51.95148351646824381, 3.976808671807906315 ) ) ;
#3592=VERTEX_POINT ( 'NONE', #5797 ) ;
#3595=CARTESIAN_POINT ( 'NONE',  ( 15.62209821594298198, 57.21425893602940249, 4.494981641845320119 ) ) ;
#3603=CARTESIAN_POINT ( 'NONE',  ( -6.743941583970623377, 63.88657993984631389, -10.82739850970073014 ) ) ;
#3608=EDGE_CURVE ( 'NONE', #5647, #567, #7819, .T. ) ;
#3612=CARTESIAN_POINT ( 'NONE',  ( 52.99999999999999289, 58.53553390593273065, -3.535533905932738197 ) ) ;
#3613=CARTESIAN_POINT ( 'NONE',  ( -61.49460156519547382, 54.99554728952567473, 0.005807220347030686396 ) ) ;
#3616=CARTESIAN_POINT ( 'NONE',  ( -26.93186442276182291, 50.75324309684062030, 2.644246209326107877 ) ) ;
#3621=CARTESIAN_POINT ( 'NONE',  ( -64.40004821475288566, 41.61990247229329043, 16.30275451258844654 ) ) ;
#3627=CARTESIAN_POINT ( 'NONE',  ( -6.785358873008338954, 67.52118754941005818, -16.88410835930674381 ) ) ;
#3630=CARTESIAN_POINT ( 'NONE',  ( 3.335481153117199060, 54.99801350816134260, -0.0001838804729987853024 ) ) ;
#3631=VECTOR ( 'NONE', #1445, 1000.000000000000000 ) ;
#3632=ORIENTED_EDGE ( 'NONE', *, *, #5230, .F. ) ;
#3633=CARTESIAN_POINT ( 'NONE',  ( 15.81093802506984858, 57.74566954809575492, 20.97791266904829044 ) ) ;
#3634=CARTESIAN_POINT ( 'NONE',  ( -8.214759031591983174, 65.81066618478850216, -18.03675305545087681 ) ) ;
#3636=CARTESIAN_POINT ( 'NONE',  ( -48.90475262238859244, 59.99999999999997158, -9.564595459368971197E-12 ) ) ;
#3642=CARTESIAN_POINT ( 'NONE',  ( -19.99785218025166600, 55.00127463874410694, 0.001534684918545882936 ) ) ;
#3643=CARTESIAN_POINT ( 'NONE',  ( -46.95981180409334854, 59.74564377627622491, -1.608358621211970263 ) ) ;
#3661=ORIENTED_EDGE ( 'NONE', *, *, #10581, .F. ) ;
#3663=CARTESIAN_POINT ( 'NONE',  ( -20.16981924998567877, 57.75067501206415699, 13.79995037456313334 ) ) ;
#3673=CARTESIAN_POINT ( 'NONE',  ( -39.90973890762001020, 55.00092042771588297, -0.009673943807180659937 ) ) ;
#3677=CARTESIAN_POINT ( 'NONE',  ( 47.00000000000000000, 55.00000000000000000, 0.000000000000000000 ) ) ;
#3678=EDGE_LOOP ( 'NONE', ( #9903, #2707, #1224, #1595, #9444, #8777 ) ) ;
#3682=CARTESIAN_POINT ( 'NONE',  ( -19.00387657603030078, 69.86840152515847535, 14.86901714484747750 ) ) ;
#3686=CARTESIAN_POINT ( 'NONE',  ( -37.18898618307433424, 44.43582214169357769, -18.32873044267784479 ) ) ;
#3687=SHAPE_REPRESENTATION_RELATIONSHIP ( 'NONE' , 'NONE' ,  #11597, #2413 ) ;
#3690=CARTESIAN_POINT ( 'NONE',  ( 18.09282150389694976, 54.98959524075147698, -0.01273383307231591190 ) ) ;
#3692=CARTESIAN_POINT ( 'NONE',  ( -29.92935756904273603, 34.87299855483264110, 6.108044681958789468 ) ) ;
#3693=CARTESIAN_POINT ( 'NONE',  ( -20.73741325422386339, 64.90628579765783002, 18.53688757488948369 ) ) ;
#3700=CARTESIAN_POINT ( 'NONE',  ( -28.57385868769931747, 55.01273333077524086, -0.01040445938396371457 ) ) ;
#3701=CARTESIAN_POINT ( 'NONE',  ( -62.13034108455730120, 51.94914922404619517, 3.974862913485895266 ) ) ;
#3714=CARTESIAN_POINT ( 'NONE',  ( 6.317087443011592640, 50.00000000000001421, -0.6593808601074064857 ) ) ;
#3716=CARTESIAN_POINT ( 'NONE',  ( 19.87282930741283948, 63.62205004655174889, 11.21167653978275958 ) ) ;
#3725=CARTESIAN_POINT ( 'NONE',  ( -50.71441498082971577, 54.99195842427500480, -0.003607703250841377916 ) ) ;
#3734=CARTESIAN_POINT ( 'NONE',  ( -65.80895658223876410, 38.19798843649414977, 12.92520887581758693 ) ) ;
#3738=CARTESIAN_POINT ( 'NONE',  ( -31.30269415623623885, 33.99224428815358579, -1.031667027462585207 ) ) ;
#3741=CARTESIAN_POINT ( 'NONE',  ( -60.73530621856283318, 48.89645762657089278, 20.10868697360108115 ) ) ;
#3742=ORIENTED_EDGE ( 'NONE', *, *, #11689, .F. ) ;
#3743=CARTESIAN_POINT ( 'NONE',  ( -13.15402772192483383, 59.74639309637463924, -1.606196551478056955 ) ) ;
#3744=CARTESIAN_POINT ( 'NONE',  ( -4.188986194789085182, 52.25407379690145859, -20.98118322582191908 ) ) ;
#3747=CARTESIAN_POINT ( 'NONE',  ( -30.78535887075297595, 34.20700043619147124, 3.085051459701278365 ) ) ;
#3748=CARTESIAN_POINT ( 'NONE',  ( -43.78535878948660098, 60.10716095388539060, -20.39140800440753054 ) ) ;
#3757=CARTESIAN_POINT ( 'NONE',  ( -54.71441367628058572, 54.99501360422757301, -0.002467102893749668121 ) ) ;
#3758=CARTESIAN_POINT ( 'NONE',  ( -45.59944951615121056, 59.24594800971062369, -2.645521645423703383 ) ) ;
#3763=CARTESIAN_POINT ( 'NONE',  ( -8.874841564931038818, 58.60437997257135834, -6.013803112307263277 ) ) ;
#3777=CARTESIAN_POINT ( 'NONE',  ( -30.66480670352544635, 40.98593724095160695, 0.0004245934155297764051 ) ) ;
#3787=CARTESIAN_POINT ( 'NONE',  ( -52.75694149779237563, 54.99300116554260853, -0.007378550177579538093 ) ) ;
#3794=FACE_OUTER_BOUND ( 'NONE', #10488, .T. ) ;
#3797=CARTESIAN_POINT ( 'NONE',  ( -19.59602372284622618, 68.34451306940553650, 16.25656885606184332 ) ) ;
#3800=CARTESIAN_POINT ( 'NONE',  ( -7.969360823174009845, 70.58422527244209732, -14.12522777056770629 ) ) ;
#3805=B_SPLINE_CURVE_WITH_KNOTS ( 'NONE', 3,
 ( #9264, #2014, #8435, #7490, #3643, #8200, #11112, #4721, #3758, #2750, #155, #3585, #8257, #8375, #6529, #6408, #9327, #2804, #2926, #7311, #10040, #6468, #11053, #1117, #9093, #6355, #2861, #7427, #33, #5446, #1834, #9984, #9151, #10097 ),
 .UNSPECIFIED., .F., .F.,
 ( 4, 2, 2, 2, 2, 2, 2, 2, 2, 2, 2, 2, 2, 2, 2, 2, 4 ),
 ( 0.02428132876980577601, 0.02579896738251766936, 0.02731660599522955923, 0.02807542530158549723, 0.02883424460794143523, 0.03035188322065331470, 0.03186952183336519417, 0.03338716044607706324, 0.03642243767150082911, 0.03794007628421271205, 0.03945771489692460193, 0.04021653420328053646, 0.04097535350963647099, 0.04249299212234831924, 0.04401063073506016055, 0.04552826934777200879, 0.04856354657319568446 ),
 .UNSPECIFIED. ) ;
#3806=CARTESIAN_POINT ( 'NONE',  ( 0.8520517685207298353, 50.51279070969081175, -2.211769638084826184 ) ) ;
#3808=CARTESIAN_POINT ( 'NONE',  ( 4.329456757236127551, 33.97246960341611555, -0.0004353087921988608999 ) ) ;
#3811=CARTESIAN_POINT ( 'NONE',  ( -54.40418125752137968, 71.24517320114661345, 13.33400169942066249 ) ) ;
#3814=CARTESIAN_POINT ( 'NONE',  ( 22.66666666666666785, 68.99999999999998579, 0.000000000000000000 ) ) ;
#3820=CARTESIAN_POINT ( 'NONE',  ( -49.57393269579290518, 54.98425279022231393, 0.004738408210547216323 ) ) ;
#3821=CARTESIAN_POINT ( 'NONE',  ( -61.54402485781515963, 52.35750010887923622, 4.247823058339725399 ) ) ;
#3823=ADVANCED_FACE ( 'NONE', ( #1987 ), #9067, .T. ) ;
#3829=CARTESIAN_POINT ( 'NONE',  ( 16.10999105973513679, 58.51886257568109784, 6.100589661946206554 ) ) ;
#3831=CARTESIAN_POINT ( 'NONE',  ( 8.058385817489730485, 34.79396711235183659, 6.140502173211014103 ) ) ;
#3841=CARTESIAN_POINT ( 'NONE',  ( -31.83648591676323392, 41.19787054414934602, -2.739720031503523945 ) ) ;
#3851=CARTESIAN_POINT ( 'NONE',  ( -35.32265116553373474, 50.16047822658878630, -1.298113203157589934 ) ) ;
#3853=CARTESIAN_POINT ( 'NONE',  ( -8.166495697937584453, 60.85006410611888583, -3.912655936626574071 ) ) ;
#3856=AXIS2_PLACEMENT_3D ( 'NONE', #9987, #5566, #1727 ) ;
#3857=DIRECTION ( 'NONE',  ( 0.000000000000000000, 0.000000000000000000, 1.000000000000000000 ) ) ;
#3858=EDGE_LOOP ( 'NONE', ( #10295, #5561, #8934 ) ) ;
#3861=VERTEX_POINT ( 'NONE', #8470 ) ;
#3863=CARTESIAN_POINT ( 'NONE',  ( 17.52230480588388417, 67.92092721363508190, 16.80419350660125843 ) ) ;
#3868=CARTESIAN_POINT ( 'NONE',  ( -48.85567157503042779, 75.97628680226326026, -2.745941867523475466 ) ) ;
#3869=SURFACE_SIDE_STYLE ('',( #8418 ) ) ;
#3870=CARTESIAN_POINT ( 'NONE',  ( -54.32961274566940801, 69.86573439484330095, 14.86481071665870601 ) ) ;
#3872=CARTESIAN_POINT ( 'NONE',  ( 47.00000000000000711, 51.46446609406725514, 3.535533905932731091 ) ) ;
#3875=CARTESIAN_POINT ( 'NONE',  ( -56.72452039520490530, 64.93179437211591676, 18.59801390061586801 ) ) ;
#3876=CARTESIAN_POINT ( 'NONE',  ( -62.45014759628331547, 49.89181376149021219, 20.39015500988638507 ) ) ;
#3881=VERTEX_POINT ( 'NONE', #4815 ) ;
#3883=CARTESIAN_POINT ( 'NONE',  ( -24.09713505895794228, 55.00123344345425380, -0.01226757850090470087 ) ) ;
#3885=DIRECTION ( 'NONE',  ( -0.04756514941544910668, 0.9988681377244376103, -0.000000000000000000 ) ) ;
#3887=CARTESIAN_POINT ( 'NONE',  ( -61.03686256008624866, 55.68802913392543275, 13.99442384959076691 ) ) ;
#3889=CARTESIAN_POINT ( 'NONE',  ( 7.506399388638331338, 34.30832474160909129, 4.109400874309620200 ) ) ;
#3892=DIRECTION ( 'NONE',  ( 1.000000000000000000, 0.000000000000000000, 0.000000000000000000 ) ) ;
#3900=CARTESIAN_POINT ( 'NONE',  ( 25.00000000000000000, 76.00000000000000000, 0.000000000000000000 ) ) ;
#3904=DIRECTION ( 'NONE',  ( 1.000000000000000000, 6.033820786006286457E-17, -0.000000000000000000 ) ) ;
#3910=CARTESIAN_POINT ( 'NONE',  ( -19.83316236458889747, 56.37610012593751208, 6.902063095245181579 ) ) ;
#3916=ORIENTED_EDGE ( 'NONE', *, *, #6143, .F. ) ;
#3918=CARTESIAN_POINT ( 'NONE',  ( -62.45014759628331547, 49.89181376149021219, 20.39015500988638507 ) ) ;
#3921=CARTESIAN_POINT ( 'NONE',  ( 34.00000000000000000, 64.99999999999998579, 0.000000000000000000 ) ) ;
#3930=CARTESIAN_POINT ( 'NONE',  ( -61.11681434411291036, 49.89209620109770071, 20.38939785324081200 ) ) ;
#3931=CARTESIAN_POINT ( 'NONE',  ( 3.998131555863420505, 40.98098423833228310, -0.0003514993523973195672 ) ) ;
#3936=DIRECTION ( 'NONE',  ( 1.000000000000000000, 6.033820786006286457E-17, -0.000000000000000000 ) ) ;
#3943=CARTESIAN_POINT ( 'NONE',  ( 11.44321751246060437, 53.17432586545520223, 6.801933848413093564 ) ) ;
#3945=CARTESIAN_POINT ( 'NONE',  ( 21.85574933723554736, 73.37275400661043534, 10.58193396047185075 ) ) ;
#3949=FACE_OUTER_BOUND ( 'NONE', #6340, .T. ) ;
#3958=CARTESIAN_POINT ( 'NONE',  ( -68.00371502632826548, 40.99428914066987062, 0.003597212120264942775 ) ) ;
#3970=CARTESIAN_POINT ( 'NONE',  ( -43.48657495774332915, 55.33066324073525521, -4.991758028738959574 ) ) ;
#3972=CARTESIAN_POINT ( 'NONE',  ( 1.556783352007605314, 50.68022262062438443, -5.615603207694791266 ) ) ;
#3975=DIRECTION ( 'NONE',  ( -1.000000000000000000, -6.033820786006286457E-17, -0.000000000000000000 ) ) ;
#3976=ADVANCED_FACE ( 'NONE', ( #10721 ), #2532, .T. ) ;
#3981=CARTESIAN_POINT ( 'NONE',  ( -42.03064326886630653, 53.96872019721284630, -20.99365203016559178 ) ) ;
#3984=CARTESIAN_POINT ( 'NONE',  ( -59.00490307935969270, 55.00061426705308065, 21.02882928537637497 ) ) ;
#3989=CARTESIAN_POINT ( 'NONE',  ( 2.790000683316907093, 50.03283139526183732, -0.6581345825051299059 ) ) ;
#3990=CARTESIAN_POINT ( 'NONE',  ( 12.14423903554155793, 49.50741477678717928, 20.43476828740966766 ) ) ;
#3991=ORIENTED_EDGE ( 'NONE', *, *, #5968, .T. ) ;
#3992=CARTESIAN_POINT ( 'NONE',  ( 10.47760422355487897, 42.10669920038468206, 16.77626177829396426 ) ) ;
#3993=CARTESIAN_POINT ( 'NONE',  ( 17.20616264586559652, 63.61741959817585013, 11.20704532413626708 ) ) ;
#3996=UNCERTAINTY_MEASURE_WITH_UNIT (LENGTH_MEASURE( 1.000000000000000082E-05 ), #1998, 'distance_accuracy_value', 'NONE');
#3999=EDGE_LOOP ( 'NONE', ( #5040, #9297, #7167, #3538, #5019, #7487, #414, #1370 ) ) ;
#4005=CARTESIAN_POINT ( 'NONE',  ( -7.999860312172237364, 57.68304994702459254, -6.476756063187334433 ) ) ;
#4007=ORIENTED_EDGE ( 'NONE', *, *, #3608, .F. ) ;
#4008=CARTESIAN_POINT ( 'NONE',  ( -41.78535879711923684, 60.10680040617825881, -20.39053309953287751 ) ) ;
#4015=ORIENTED_EDGE ( 'NONE', *, *, #48, .F. ) ;
#4020=CARTESIAN_POINT ( 'NONE',  ( -38.83024551010986869, 52.26031083538927646, -13.79250609426764385 ) ) ;
#4029=CARTESIAN_POINT ( 'NONE',  ( -38.04614405021798262, 51.23507084643394194, -3.306421959314382875 ) ) ;
#4031=CARTESIAN_POINT ( 'NONE',  ( -4.375366960226389601, 57.35780173001101900, -6.590899248362319440 ) ) ;
#4041=CARTESIAN_POINT ( 'NONE',  ( -64.51030549024622474, 43.28227691760346119, 17.55408017169854418 ) ) ;
#4046=CARTESIAN_POINT ( 'NONE',  ( -60.45014771802851072, 49.89223742090062075, 20.38901927491476584 ) ) ;
#4048=CIRCLE ( 'NONE', #10725, 4.999999999999990230 ) ;
#4055=CARTESIAN_POINT ( 'NONE',  ( -19.88142569839470042, 67.52672413929985851, 16.89011978890229315 ) ) ;
#4056=ORIENTED_EDGE ( 'NONE', *, *, #8254, .F. ) ;
#4058=CARTESIAN_POINT ( 'NONE',  ( -8.404080175971420985, 68.33445312550857409, -16.24552120034004332 ) ) ;
#4059=CARTESIAN_POINT ( 'NONE',  ( -29.83024526348565431, 43.30463061081272969, 7.809786529886623363 ) ) ;
#4061=DIRECTION ( 'NONE',  ( 0.000000000000000000, 1.000000000000000000, 0.000000000000000000 ) ) ;
#4067=CARTESIAN_POINT ( 'NONE',  ( 52.99999999999999289, 55.00000000000000000, 0.000000000000000000 ) ) ;
#4068=CARTESIAN_POINT ( 'NONE',  ( -33.95794589294774823, 47.99441920491325675, -0.3443687011034463619 ) ) ;
#4070=CARTESIAN_POINT ( 'NONE',  ( -11.52239577449127061, 75.97627689174807131, -2.745668057393931161 ) ) ;
#4071=CARTESIAN_POINT ( 'NONE',  ( -52.42856357389445066, 59.99999999999997158, -5.034386850915387018E-15 ) ) ;
#4078=CARTESIAN_POINT ( 'NONE',  ( 16.47760469315713294, 57.74566955740679930, 20.97627666568605420 ) ) ;
#4085=CARTESIAN_POINT ( 'NONE',  ( -49.31852470631967122, 59.33770604155814254, -2.508136721262845370 ) ) ;
#4087=CARTESIAN_POINT ( 'NONE',  ( 13.22345001879655335, 51.46496636567017191, 6.139952220504262037 ) ) ;
#4090=CARTESIAN_POINT ( 'NONE',  ( 47.00000000000000000, 55.00000000000000000, 0.000000000000000000 ) ) ;
#4104=CARTESIAN_POINT ( 'NONE',  ( -9.969360172258976860, 70.58303384883494402, -14.12411716821732277 ) ) ;
#4106=CARTESIAN_POINT ( 'NONE',  ( -10.17314267936212069, 72.54319253558377056, -11.73149487979574168 ) ) ;
#4107=CARTESIAN_POINT ( 'NONE',  ( -35.07137196547176927, 41.55265658068579171, -4.083739209675547599 ) ) ;
#4109=CARTESIAN_POINT ( 'NONE',  ( 36.99999999999999289, 50.00000000000001421, 6.123233995736750505E-16 ) ) ;
#4110=CARTESIAN_POINT ( 'NONE',  ( -15.48546139901933572, 59.99999999999970157, 0.3308755477335553197 ) ) ;
#4117=CARTESIAN_POINT ( 'NONE',  ( -45.33346893179080439, 57.68097894510658108, -6.473283064943208487 ) ) ;
#4120=CARTESIAN_POINT ( 'NONE',  ( -39.16026728571524984, 50.89059911655681390, -20.69167526169209026 ) ) ;
#4129=LINE ( 'NONE', #6786, #215 ) ;
#4131=CARTESIAN_POINT ( 'NONE',  ( 0.1442708919848544047, 44.43605983923426805, -18.32883121229183487 ) ) ;
#4141=CARTESIAN_POINT ( 'NONE',  ( -48.54021952654307626, 58.97499403197477363, -3.050551747025779914 ) ) ;
#4143=CARTESIAN_POINT ( 'NONE',  ( -61.83316972777281961, 51.09090217642938114, 5.855680158205122332 ) ) ;
#4150=AXIS2_PLACEMENT_3D ( 'NONE', #10387, #9313, #2968 ) ;
#4156=CARTESIAN_POINT ( 'NONE',  ( -14.23626113480177935, 55.01767704715457796, 0.008670778123901936099 ) ) ;
#4158=CIRCLE ( 'NONE', #8574, 4.999999999999997335 ) ;
#4160=EDGE_LOOP ( 'NONE', ( #6165, #5954, #3510, #4606, #5896, #5396, #8610, #1534 ) ) ;
#4163=CARTESIAN_POINT ( 'NONE',  ( -17.82693376281896391, 72.53768310958322729, 11.72612467905221934 ) ) ;
#4165=CARTESIAN_POINT ( 'NONE',  ( -62.30250798370089882, 46.00592899164083605, 19.01213062829916112 ) ) ;
#4166=CARTESIAN_POINT ( 'NONE',  ( -21.07727389599352819, 61.60348718499724896, 12.35586511164976287 ) ) ;
#4170=CARTESIAN_POINT ( 'NONE',  ( -27.54087155171534462, 52.49442175028256230, 4.339376312279030756 ) ) ;
#4176=VECTOR ( 'NONE', #4380, 1000.000000000000000 ) ;
#4179=CARTESIAN_POINT ( 'NONE',  ( -42.70869921250305623, 54.65600185176862880, -6.994195710570620506 ) ) ;
#4181=CARTESIAN_POINT ( 'NONE',  ( -54.63607242817042930, 69.12530316040908929, 15.58420556269393309 ) ) ;
#4182=CARTESIAN_POINT ( 'NONE',  ( 12.14423903554155793, 49.50741477678717928, 20.43476828740966766 ) ) ;
#4191=DIRECTION ( 'NONE',  ( 1.000000000000000000, 6.033820786006286457E-17, -0.000000000000000000 ) ) ;
#4194=CARTESIAN_POINT ( 'NONE',  ( -20.50647613538409075, 59.12524989819403487, 20.69783765389080799 ) ) ;
#4207=CARTESIAN_POINT ( 'NONE',  ( -55.41760771481728653, 58.30620755303042557, 6.186168293415320818 ) ) ;
#4219=CARTESIAN_POINT ( 'NONE',  ( -4.047728495240956903, 54.99641480296497775, 0.008019458024605742932 ) ) ;
#4223=VERTEX_POINT ( 'NONE', #11852 ) ;
#4228=CARTESIAN_POINT ( 'NONE',  ( -50.85567158358731632, 75.98119253013058483, -2.745941642920928683 ) ) ;
#4230=CARTESIAN_POINT ( 'NONE',  ( -61.21370359292568253, 51.91450527571464590, 20.80059449010516204 ) ) ;
#4231=CARTESIAN_POINT ( 'NONE',  ( -33.63031969913447483, 40.99414563559565039, -0.6879892896588567508 ) ) ;
#4237=CARTESIAN_POINT ( 'NONE',  ( 14.14423903981857755, 49.50929293985068114, 20.43023407247793699 ) ) ;
#4241=CARTESIAN_POINT ( 'NONE',  ( -23.16649539194673935, 56.37547255868592799, 6.900582075605663057 ) ) ;
#4243=CARTESIAN_POINT ( 'NONE',  ( -44.39182476880109363, 68.38060868816502591, -16.29271878486493463 ) ) ;
#4244=CARTESIAN_POINT ( 'NONE',  ( 12.85570563148687739, 52.25434904275299175, 21.01882863504484789 ) ) ;
#4254=CARTESIAN_POINT ( 'NONE',  ( -29.54809237377008202, 34.60091625530366599, 5.109976345715927515 ) ) ;
#4260=CARTESIAN_POINT ( 'NONE',  ( -21.32947787934852357, 63.04568470447853912, 19.42265540296757464 ) ) ;
#4267=ORIENTED_EDGE ( 'NONE', *, *, #1808, .T. ) ;
#4269=CARTESIAN_POINT ( 'NONE',  ( -29.45858744683659936, 48.07282909709525853, 1.028500488243905719 ) ) ;
#4279=CARTESIAN_POINT ( 'NONE',  ( 19.75947799528538340, 54.99150360729431952, -0.02481536840781081721 ) ) ;
#4285=CARTESIAN_POINT ( 'NONE',  ( -9.662811212962280294, 69.86524355530642083, -14.86597185903763219 ) ) ;
#4287=CARTESIAN_POINT ( 'NONE',  ( -47.14426297200904514, 71.80510559133185211, -12.92232144701529428 ) ) ;
#4288=CARTESIAN_POINT ( 'NONE',  ( -36.46040627036565951, 42.74970947531311793, -7.056004382930415098 ) ) ;
#4292=CARTESIAN_POINT ( 'NONE',  ( 6.329456780446692576, 33.97189653527247089, -0.0004287163746460355418 ) ) ;
#4296=CARTESIAN_POINT ( 'NONE',  ( -30.16689009792652243, 49.15416857633141490, 3.904260228111898989 ) ) ;
#4298=CARTESIAN_POINT ( 'NONE',  ( 21.18908267236805898, 73.37124140341018119, 10.58130724700091463 ) ) ;
#4300=CARTESIAN_POINT ( 'NONE',  ( 9.810937555461070048, 42.10554236623130464, 16.77741859935663626 ) ) ;
#4307=CARTESIAN_POINT ( 'NONE',  ( -66.79101289578984790, 50.03300633731364400, 0.6594954161248131053 ) ) ;
#4309=CARTESIAN_POINT ( 'NONE',  ( -2.188986190505546769, 52.25407376895000056, -20.97627476078892528 ) ) ;
#4312=CARTESIAN_POINT ( 'NONE',  ( -52.42856357389445066, 59.99999999999997158, -5.034386850915387018E-15 ) ) ;
#4316=STYLED_ITEM('',(#11895),#684);
#4317=CARTESIAN_POINT ( 'NONE',  ( -44.07074648197151845, 61.10275710191199749, -20.11236068975357938 ) ) ;
#4325=CARTESIAN_POINT ( 'NONE',  ( -36.55667896093988389, 51.48427161832111665, -6.093033236249906004 ) ) ;
#4343=CARTESIAN_POINT ( 'NONE',  ( 22.09282151157359309, 54.98265345718393604, -0.01967570506841854680 ) ) ;
#4350=CARTESIAN_POINT ( 'NONE',  ( -55.45210586135002728, 71.88485191958531573, 12.52183031059725771 ) ) ;
#4352=CARTESIAN_POINT ( 'NONE',  ( -28.82693382303331475, 37.45538988585808937, 11.71519277693090366 ) ) ;
#4353=CARTESIAN_POINT ( 'NONE',  ( -45.29698632460738139, 60.99542764961179842, -12.67644002407605086 ) ) ;
#4359=CARTESIAN_POINT ( 'NONE',  ( 4.881307793505825110, 34.60946683332392126, -5.106800360247272685 ) ) ;
#4361=CARTESIAN_POINT ( 'NONE',  ( 8.654567787479487961, 50.16095913586803334, 1.299965765103639148 ) ) ;
#4362=CARTESIAN_POINT ( 'NONE',  ( 11.90727647329997829, 54.99834172827340240, 0.01637095017119612195 ) ) ;
#4365=CARTESIAN_POINT ( 'NONE',  ( -67.52720549794999272, 34.02364409886038743, 2.748840581154547102 ) ) ;
#4368=DIRECTION ( 'NONE',  ( 1.000000000000000000, 6.033820786006286457E-17, -0.000000000000000000 ) ) ;
#4375=CARTESIAN_POINT ( 'NONE',  ( -55.50627899214600092, 66.73177265193905328, 17.54361557889675893 ) ) ;
#4380=DIRECTION ( 'NONE',  ( 1.000000000000000000, 6.033820786006286457E-17, -0.000000000000000000 ) ) ;
#4384=ORIENTED_EDGE ( 'NONE', *, *, #4529, .F. ) ;
#4389=CARTESIAN_POINT ( 'NONE',  ( 9.793834090903223100, 42.78911815673161811, 7.039953125326757544 ) ) ;
#4395=AXIS2_PLACEMENT_3D ( 'NONE', #5551, #207, #1103 ) ;
#4396=ORIENTED_EDGE ( 'NONE', *, *, #10917, .F. ) ;
#4401=DIRECTION ( 'NONE',  ( -1.000000000000000000, -6.033820786006286457E-17, -0.000000000000000000 ) ) ;
#4408=CARTESIAN_POINT ( 'NONE',  ( -18.18548385789268451, 57.21583455123535344, 4.494158473437730450 ) ) ;
#4409=EDGE_CURVE ( 'NONE', #1675, #3592, #4048, .T. ) ;
#4412=CARTESIAN_POINT ( 'NONE',  ( -34.05849041764468410, 34.82468742385552218, -6.128056420806536231 ) ) ;
#4421=CARTESIAN_POINT ( 'NONE',  ( 14.48524493375191291, 53.39293360022251278, 4.746189266409619023 ) ) ;
#4422=CARTESIAN_POINT ( 'NONE',  ( -57.29127706180261725, 59.71020960438666236, 5.197211960637448058 ) ) ;
#4424=CARTESIAN_POINT ( 'NONE',  ( 18.85563813666183819, 67.92324243781868631, 16.80650911442449313 ) ) ;
#4426=CARTESIAN_POINT ( 'NONE',  ( -9.662811212962280294, 69.86524355530642083, -14.86597185903763219 ) ) ;
#4431=DIRECTION ( 'NONE',  ( 0.9999998346844722885, -0.0005712585774195265247, 6.553370117834432030E-05 ) ) ;
#4434=CARTESIAN_POINT ( 'NONE',  ( -41.78535879711923684, 60.10680040617825881, -20.39053309953287751 ) ) ;
#4439=CARTESIAN_POINT ( 'NONE',  ( -60.20667922569305830, 56.29624695176077864, 4.839977866460043465 ) ) ;
#4440=ORIENTED_EDGE ( 'NONE', *, *, #10537, .T. ) ;
#4450=CARTESIAN_POINT ( 'NONE',  ( 0.4815530525298790665, 52.78317629943902034, -4.493698677454305290 ) ) ;
#4451=CARTESIAN_POINT ( 'NONE',  ( -22.12707294284022197, 53.16908462427974769, 14.02455705437751909 ) ) ;
#4457=ADVANCED_FACE ( 'NONE', ( #5949 ), #9642, .T. ) ;
#4462=CARTESIAN_POINT ( 'NONE',  ( -22.24059675286479276, 55.01153819220757413, -0.02355272863444527257 ) ) ;
#4467=CARTESIAN_POINT ( 'NONE',  ( -59.82750509709391196, 59.10995506582904824, 20.69284243654335498 ) ) ;
#4469=CARTESIAN_POINT ( 'NONE',  ( -56.83961221553562382, 66.73132451083796468, 17.54318035443342438 ) ) ;
#4473=CARTESIAN_POINT ( 'NONE',  ( -5.929357825456832209, 64.91315550346766372, -18.55154749960842153 ) ) ;
#4476=CARTESIAN_POINT ( 'NONE',  ( -5.240525354424131699, 54.99835323915754515, 0.01636088839724062979 ) ) ;
#4478=CARTESIAN_POINT ( 'NONE',  ( 9.522371807443699154, 38.19365890154983845, 12.92340179382780896 ) ) ;
#4479=CARTESIAN_POINT ( 'NONE',  ( -6.160267096003628318, 59.12214581854949103, -20.69010011304746044 ) ) ;
#4481=CYLINDRICAL_SURFACE ( 'NONE', #2473, 4.999999999999984013 ) ;
#4503=CARTESIAN_POINT ( 'NONE',  ( 4.922725082627545490, 41.59604121305380886, -4.066663295143957413 ) ) ;
#4511=ORIENTED_EDGE ( 'NONE', *, *, #9828, .F. ) ;
#4513=CARTESIAN_POINT ( 'NONE',  ( -52.46182469558537775, 54.99624011979340565, -0.004044406450102152988 ) ) ;
#4517=CARTESIAN_POINT ( 'NONE',  ( -11.57142270279487306, 60.00000000000001421, -4.065933922700817035E-15 ) ) ;
#4519=CARTESIAN_POINT ( 'NONE',  ( -66.47562283042974229, 38.19906477560226676, 12.92409071120044040 ) ) ;
#4522=CARTESIAN_POINT ( 'NONE',  ( -11.39182375260447166, 73.60042400440836730, -9.933379572949093017 ) ) ;
#4528=CARTESIAN_POINT ( 'NONE',  ( -30.11869220662914159, 34.20731585996448132, 3.085050890631813036 ) ) ;
#4529=EDGE_CURVE ( 'NONE', #7593, #9403, #6357, .T. ) ;
#4532=CARTESIAN_POINT ( 'NONE',  ( 15.75947798662055988, 54.99526034255116258, -0.01574567900935226750 ) ) ;
#4534=CARTESIAN_POINT ( 'NONE',  ( 24.33333333333332149, 76.00000000000000000, 0.000000000000000000 ) ) ;
#4536=CARTESIAN_POINT ( 'NONE',  ( -15.14429485721040614, 76.01882847486140804, 2.745652427074330326 ) ) ;
#4538=CARTESIAN_POINT ( 'NONE',  ( 63.00000000000000000, 55.00000000000000000, 2.445500000000003116 ) ) ;
#4543=DIRECTION ( 'NONE',  ( 6.527513432760042190E-05, -0.0004526335343839516683, -0.9999998954310147514 ) ) ;
#4544=CARTESIAN_POINT ( 'NONE',  ( -32.24307070243303741, 54.99420864160337885, 0.001526422163665167291 ) ) ;
#4545=PRODUCT_DEFINITION ( 'UNKNOWN', '', #5096, #8822 ) ;
#4546=CARTESIAN_POINT ( 'NONE',  ( -50.84658144432280125, 59.74596735251822821, 1.607341111116408428 ) ) ;
#4550=CARTESIAN_POINT ( 'NONE',  ( -56.71072052760479920, 58.76569921069902591, 3.305499569647178060 ) ) ;
#4551=VERTEX_POINT ( 'NONE', #2805 ) ;
#4564=CARTESIAN_POINT ( 'NONE',  ( -5.878133643754496873, 62.20801019244017027, -12.02644650578262997 ) ) ;
#4565=ADVANCED_FACE ( 'NONE', ( #8201 ), #1898, .T. ) ;
#4573=CARTESIAN_POINT ( 'NONE',  ( -40.79520177461022001, 54.99765425461028912, 0.005074365896716425024 ) ) ;
#4580=CARTESIAN_POINT ( 'NONE',  ( -17.27494751259140315, 73.62640980466187557, 9.944421848179040069 ) ) ;
#4585=CARTESIAN_POINT ( 'NONE',  ( -32.72515708217407138, 34.82695427582095959, -6.127117481167428714 ) ) ;
#4586=PRESENTATION_STYLE_ASSIGNMENT (( #10080 ) ) ;
#4589=CARTESIAN_POINT ( 'NONE',  ( -67.88985479635340425, 48.90596771384532815, 3.517032652760510913 ) ) ;
#4591=CARTESIAN_POINT ( 'NONE',  ( -41.88142568112290576, 58.08538812386944983, -20.80148275009198855 ) ) ;
#4592=CARTESIAN_POINT ( 'NONE',  ( 0.2748429140369315071, 38.70467982241823535, -13.38321124372595783 ) ) ;
#4599=CARTESIAN_POINT ( 'NONE',  ( -41.56959446453805640, 54.99645083705581072, -0.01182256036410916228 ) ) ;
#4600=CARTESIAN_POINT ( 'NONE',  ( -57.45740457225677034, 55.65951194273775826, 4.966982812372184419 ) ) ;
#4602=ADVANCED_FACE ( 'NONE', ( #10098 ), #7366, .T. ) ;
#4606=ORIENTED_EDGE ( 'NONE', *, *, #11689, .T. ) ;
#4607=CARTESIAN_POINT ( 'NONE',  ( 17.18896242946999919, 60.50854855881860317, 20.47421955154796436 ) ) ;
#4610=CARTESIAN_POINT ( 'NONE',  ( 12.12266132830104226, 54.34318581670489579, 4.967339324998079064 ) ) ;
#4615=AXIS2_PLACEMENT_3D ( 'NONE', #10964, #9957, #6497 ) ;
#4617=CARTESIAN_POINT ( 'NONE',  ( 5.544577452450643484, 50.12720890011707553, -1.300076040883277884 ) ) ;
#4618=CARTESIAN_POINT ( 'NONE',  ( 4.335193296466895774, 42.05253176472596977, -5.362557364853363318 ) ) ;
#4631=CARTESIAN_POINT ( 'NONE',  ( -28.53821618333067534, 54.99572319873755788, 0.001494283935380159292 ) ) ;
#4632=SHAPE_DEFINITION_REPRESENTATION ( #3566, #11597 ) ;
#4637=CARTESIAN_POINT ( 'NONE',  ( 7.485949637387768085, 50.00826809906988757, 0.3311691434445088178 ) ) ;
#4640=CARTESIAN_POINT ( 'NONE',  ( 0.8268573817076104726, 37.44832105976551873, -11.71822709476406210 ) ) ;
#4644=CARTESIAN_POINT ( 'NONE',  ( -8.839809468419982608, 72.54364378520992318, -11.73195350307014273 ) ) ;
#4647=CARTESIAN_POINT ( 'NONE',  ( -10.81689418260944180, 58.76766599462401786, -3.303253631844218940 ) ) ;
#4650=CARTESIAN_POINT ( 'NONE',  ( -52.36394100382401717, 74.78921131832989033, 7.080786878544920171 ) ) ;
#4651=CARTESIAN_POINT ( 'NONE',  ( -5.608280846031337141, 57.05942937149918492, -21.01412426850803783 ) ) ;
#4653=CARTESIAN_POINT ( 'NONE',  ( 22.23809523809524435, 59.99999999999998579, 0.000000000000000000 ) ) ;
#4657=CARTESIAN_POINT ( 'NONE',  ( -33.12853505168487089, 55.00369317299735172, 0.0002287014689915395241 ) ) ;
#4658=CARTESIAN_POINT ( 'NONE',  ( -55.51934695731827674, 57.21273593182136352, 4.486748991334322589 ) ) ;
#4661=CARTESIAN_POINT ( 'NONE',  ( -58.40439726469009685, 61.62069348438144800, 12.39615534886321235 ) ) ;
#4663=CARTESIAN_POINT ( 'NONE',  ( -6.214759040711413718, 65.81103152010582846, -18.03762937187994453 ) ) ;
#4667=CARTESIAN_POINT ( 'NONE',  ( 3.571755578639977724, 50.00000000000001421, 2.874253840576960811E-12 ) ) ;
#4670=VERTEX_POINT ( 'NONE', #3588 ) ;
#4674=CARTESIAN_POINT ( 'NONE',  ( -52.25615635136895776, 67.37056480795911284, 6.610292622630669079 ) ) ;
#4685=CARTESIAN_POINT ( 'NONE',  ( -56.23628154728545780, 55.00641776599200483, 0.01848975112542444732 ) ) ;
#4692=FACE_OUTER_BOUND ( 'NONE', #11736, .T. ) ;
#4697=CARTESIAN_POINT ( 'NONE',  ( 14.47760468889531182, 57.74566952947367326, 20.98118467575540436 ) ) ;
#4704=CARTESIAN_POINT ( 'NONE',  ( -36.47762819585614835, 42.07544065584382764, -16.80749884933775462 ) ) ;
#4705=CARTESIAN_POINT ( 'NONE',  ( -56.05785376386896246, 64.93131079446247611, 18.59685268580366468 ) ) ;
#4708=CARTESIAN_POINT ( 'NONE',  ( 0.4609857007025546793, 50.66760339081043441, -2.501461926089155074 ) ) ;
#4709=CARTESIAN_POINT ( 'NONE',  ( 8.189038476963473201, 38.19597440261895827, 12.92108669627241646 ) ) ;
#4712=CARTESIAN_POINT ( 'NONE',  ( -47.18905769862622890, 73.33034157825031230, -10.56456148164999398 ) ) ;
#4713=CARTESIAN_POINT ( 'NONE',  ( -64.51030549024622474, 43.28227691760346119, 17.55408017169854418 ) ) ;
#4720=CARTESIAN_POINT ( 'NONE',  ( -21.46186838525607499, 54.99879797654112679, -0.003499567500229079815 ) ) ;
#4721=CARTESIAN_POINT ( 'NONE',  ( -45.79623854691614326, 59.33124940395137514, -2.503488177144706395 ) ) ;
#4725=CARTESIAN_POINT ( 'NONE',  ( 22.33333333333333570, 61.99999999999997868, 0.000000000000000000 ) ) ;
#4738=AXIS2_PLACEMENT_3D ( 'NONE', #6164, #8011, #1383 ) ;
#4739=CARTESIAN_POINT ( 'NONE',  ( -41.45530645628071653, 58.40375168898731317, -13.59199727772139710 ) ) ;
#4749=CARTESIAN_POINT ( 'NONE',  ( -34.15346748487235828, 50.00825927070384580, -0.3308703489901499428 ) ) ;
#4751=CARTESIAN_POINT ( 'NONE',  ( 4.375386355529371052, 48.65700148509509404, -3.000201103635157018 ) ) ;
#4759=CARTESIAN_POINT ( 'NONE',  ( -9.662811212962280294, 69.86524355530642083, -14.86597185903763219 ) ) ;
#4762=CARTESIAN_POINT ( 'NONE',  ( -43.83980969374544401, 66.71858909844225138, -17.55257377017560216 ) ) ;
#4763=CARTESIAN_POINT ( 'NONE',  ( -51.69727455458300369, 74.78870212167194609, 7.080596778485133136 ) ) ;
#4764=ORIENTED_EDGE ( 'NONE', *, *, #869, .T. ) ;
#4766=EDGE_CURVE ( 'NONE', #3266, #1626, #8556, .T. ) ;
#4767=CARTESIAN_POINT ( 'NONE',  ( -3.044769863957841327, 52.78589301970062309, -4.495079137651556422 ) ) ;
#4768=CARTESIAN_POINT ( 'NONE',  ( 5.506399570602333426, 34.30736306936326230, 4.109392375493936100 ) ) ;
#4770=CARTESIAN_POINT ( 'NONE',  ( -43.63602718628743560, 63.99223089048333435, -19.01333957068342428 ) ) ;
#4771=CARTESIAN_POINT ( 'NONE',  ( -58.05785365788000263, 64.93276152744238061, 18.60033633024681521 ) ) ;
#4780=CARTESIAN_POINT ( 'NONE',  ( -22.33546444871533154, 54.99950364521073709, -0.001766467382170159531 ) ) ;
#4781=CARTESIAN_POINT ( 'NONE',  ( -48.90475262238859244, 59.99999999999997158, -9.564595459368971197E-12 ) ) ;
#4786=CARTESIAN_POINT ( 'NONE',  ( -59.59524304407526074, 59.09388748838112093, 13.47225211819516666 ) ) ;
#4788=CARTESIAN_POINT ( 'NONE',  ( -3.608280849245335542, 57.05942974268126022, -21.01780866629736977 ) ) ;
#4791=CYLINDRICAL_SURFACE ( 'NONE', #1022, 2.999999999999999112 ) ;
#4793=B_SPLINE_CURVE_WITH_KNOTS ( 'NONE', 3,
 ( #4312, #6243, #9933, #11782, #10708, #7257, #6360, #5336, #4550, #8202, #9043, #1556, #2522, #2633, #4439, #820, #1667, #3411, #8143, #10826, #9988, #3349, #6187, #3590, #5222, #8870, #10884, #7971, #11607, #8925, #2695, #1782, #5449, #7022 ),
 .UNSPECIFIED., .F., .F.,
 ( 4, 2, 2, 2, 2, 2, 2, 2, 2, 2, 2, 2, 2, 2, 2, 2, 4 ),
 ( 0.09713928911131490540, 0.09865623822481217609, 0.1001731873383094468, 0.1016901364518067175, 0.1032070855653039881, 0.1047240346788012588, 0.1062409837922985295, 0.1077579329057958002, 0.1092748820192930709, 0.1107918311327903138, 0.1123087802462875706, 0.1138257293597848274, 0.1153426784732820842, 0.1168596275867793410, 0.1183765767002765978, 0.1198935258137738408, 0.1214104749272710976 ),
 .UNSPECIFIED. ) ;
#4796=ORIENTED_EDGE ( 'NONE', *, *, #7193, .F. ) ;
#4800=CARTESIAN_POINT ( 'NONE',  ( -39.70300543809604221, 54.31243699202812536, -13.99175817854623816 ) ) ;
#4803=EDGE_CURVE ( 'NONE', #8948, #1817, #1960, .T. ) ;
#4812=DIRECTION ( 'NONE',  ( -1.000000000000000000, -6.033820786006286457E-17, 0.000000000000000000 ) ) ;
#4813=DIRECTION ( 'NONE',  ( 0.000000000000000000, 1.000000000000000000, 0.000000000000000000 ) ) ;
#4814=CARTESIAN_POINT ( 'NONE',  ( -17.79192078018706624, 58.60112408783383131, 6.006281318062062446 ) ) ;
#4815=CARTESIAN_POINT ( 'NONE',  ( 62.44550000000000267, 55.00000000000000000, 2.999999999999995559 ) ) ;
#4824=CARTESIAN_POINT ( 'NONE',  ( -56.63607177307330431, 69.12418599258134577, 15.58301102096070245 ) ) ;
#4834=CARTESIAN_POINT ( 'NONE',  ( -9.069501975036009966, 57.64327492203570102, -4.247356385754962105 ) ) ;
#4837=CARTESIAN_POINT ( 'NONE',  ( -51.49358338236809374, 75.68949746983442139, 4.121906040642151936 ) ) ;
#4838=CARTESIAN_POINT ( 'NONE',  ( 19.53960773325150768, 67.25030761837875559, 7.055968998884240229 ) ) ;
#4846=CARTESIAN_POINT ( 'NONE',  ( -60.83651074932581082, 55.00008616263955474, -0.003570840406533045113 ) ) ;
#4848=ADVANCED_FACE ( 'NONE', ( #4965 ), #5030, .T. ) ;
#4849=DIRECTION ( 'NONE',  ( 0.000000000000000000, 0.000000000000000000, -1.000000000000000000 ) ) ;
#4851=CARTESIAN_POINT ( 'NONE',  ( 2.208079232538515679, 48.20508033090954569, -1.701303895902414709 ) ) ;
#4853=CARTESIAN_POINT ( 'NONE',  ( -5.030643890195627854, 62.08057558410310861, -19.78873666113293694 ) ) ;
#4864=CARTESIAN_POINT ( 'NONE',  ( 23.47754340821147068, 75.43020022661498558, 5.490793176664390707 ) ) ;
#4874=CARTESIAN_POINT ( 'NONE',  ( 10.10998770594448359, 48.90696675832015927, 3.515728384091711511 ) ) ;
#4881=CARTESIAN_POINT ( 'NONE',  ( -62.73530513678402087, 48.89572068339310107, 20.11073150603193938 ) ) ;
#4882=DIRECTION ( 'NONE',  ( -0.7071067811865519026, 0.000000000000000000, 0.7071067811865431318 ) ) ;
#4889=CARTESIAN_POINT ( 'NONE',  ( 2.013601557404307574, 50.16004720627262969, -1.296442066224429146 ) ) ;
#4891=CARTESIAN_POINT ( 'NONE',  ( 47.00000000000000000, 60.00000000000000000, 6.123233995736769241E-16 ) ) ;
#4893=CARTESIAN_POINT ( 'NONE',  ( 20.52241600750495820, 73.36972880021862409, 10.58068053353214566 ) ) ;
#4894=CARTESIAN_POINT ( 'NONE',  ( 5.169754736345680612, 41.20621168070887563, 2.739677827818288947 ) ) ;
#4898=CARTESIAN_POINT ( 'NONE',  ( -19.37797842336306431, 58.76497942189116941, 3.306305682627446618 ) ) ;
#4908=CARTESIAN_POINT ( 'NONE',  ( 7.556752435464094475, 49.39015905361354442, 4.313964523666476758 ) ) ;
#4910=CARTESIAN_POINT ( 'NONE',  ( -34.85572910849313644, 38.22605186251247744, -12.89098713163435228 ) ) ;
#4922=CARTESIAN_POINT ( 'NONE',  ( -51.36965469666524342, 68.18978755587353646, 4.719195284573421745 ) ) ;
#4932=CARTESIAN_POINT ( 'NONE',  ( -50.48899989085627027, 59.74688460148684754, -1.604905836750670778 ) ) ;
#4935=CARTESIAN_POINT ( 'NONE',  ( -6.125254113511556575, 59.17098985002619571, -5.625509189411977751 ) ) ;
#4939=ORIENTED_EDGE ( 'NONE', *, *, #5200, .F. ) ;
#4943=CARTESIAN_POINT ( 'NONE',  ( -63.63584090060282961, 46.00639722032484968, 19.01118640546643590 ) ) ;
#4947=CARTESIAN_POINT ( 'NONE',  ( -71.09399662003431786, 50.00000004634800632, -0.0006807936302138478625 ) ) ;
#4948=CARTESIAN_POINT ( 'NONE',  ( -62.51030605291772702, 43.28161195024001273, 17.55542603392786916 ) ) ;
#4953=CARTESIAN_POINT ( 'NONE',  ( -15.14429485721040614, 76.01882847486140804, 2.745652427074330326 ) ) ;
#4955=CARTESIAN_POINT ( 'NONE',  ( -4.941614180435440318, 57.05942949522437146, -21.01535240110448299 ) ) ;
#4956=CARTESIAN_POINT ( 'NONE',  ( -27.12710454428388118, 47.94392800691067436, 12.25026322333570228 ) ) ;
#4957=FACE_OUTER_BOUND ( 'NONE', #7189, .T. ) ;
#4964=CARTESIAN_POINT ( 'NONE',  ( -62.57658715170816066, 54.99925176542368632, 0.005738867717030676080 ) ) ;
#4965=FACE_OUTER_BOUND ( 'NONE', #3678, .T. ) ;
#4966=CIRCLE ( 'NONE', #8299, 4.999999999999997335 ) ;
#4969=CARTESIAN_POINT ( 'NONE',  ( -16.55667896787908333, 61.80197853705212907, 1.825560432032844460 ) ) ;
#4970=AXIS2_PLACEMENT_3D ( 'NONE', #8670, #2310, #4061 ) ;
#4972=CARTESIAN_POINT ( 'NONE',  ( -19.63602748969081446, 62.08618401115764129, 19.80343740535094099 ) ) ;
#4982=DIRECTION ( 'NONE',  ( -1.000000000000000000, -6.033820786006286457E-17, -0.000000000000000000 ) ) ;
#4984=CARTESIAN_POINT ( 'NONE',  ( -5.337209886265139147, 63.04750289227570192, -19.42727033598380970 ) ) ;
#4987=DIRECTION ( 'NONE',  ( 1.000000000000000000, 6.033820786006286457E-17, -0.000000000000000000 ) ) ;
#4992=CARTESIAN_POINT ( 'NONE',  ( 25.00000000000000000, 76.00000000000000000, 0.000000000000000000 ) ) ;
#4995=CARTESIAN_POINT ( 'NONE',  ( 6.417054786244230868, 48.01588556897357307, -0.6870108247934131329 ) ) ;
#4999=B_SPLINE_SURFACE_WITH_KNOTS ( 'NONE', 3, 3, ( 
 ( #8681, #11413, #3223, #2328, #637, #7008, #5998, #9632, #1427, #4244, #4182, #7843, #4300, #2445, #11472, #3283, #6953, #10578, #2379, #2682, #7303, #9086, #9200, #5322, #9143, #5494, #4592, #6229, #2794, #8975, #751, #4651, #4479, #10869, #925, #810, #3634, #864, #8131, #4426, #11656, #8249, #990, #3466, #25, #4536, #11769, #6288, #7131, #6460, #10088, #10932, #2562, #8083, #3693, #11827, #3577, #6348, #10982, #7247, #1886, #5556, #8191, #11716, #9977, #9860, #9919, #1717, #1825, #7357, #10031, #10753, #2742, #6401, #1654, #3516, #1772, #7185, #10810, #2620, #5383, #9033, #5438, #11044, #1290, #3748, #10334, #9319, #8304, #5804, #2852, #7482, #11104, #1048, #5741, #7416, #8427, #8546, #10272, #11286, #6521, #9258, #10151, #2132, #3100, #1950, #4771, #5619, #6765, #6640, #212, #329, #7653, #3876, #2918, #6583, #8490, #4713, #9377, #8365, #2070, #85, #7537, #146 ),
 ( #3814, #10213, #1171, #4838, #5860, #3993, #6704, #268, #2006, #11159, #9438, #5678, #1227, #10392, #1107, #7595, #4894, #2974, #3931, #11225, #2188, #9499, #3034, #8613, #9729, #6995, #9676, #2248, #10446, #390, #11459, #1355, #11580, #2429, #3268, #7890, #7827, #11521, #3327, #5917, #6939, #564, #2368, #2492, #9562, #6097, #10618, #1529, #11344, #7946, #5022, #8669, #9792, #9620, #4166, #5193, #5986, #8783, #6040, #1415, #450, #4956, #8845, #6157, #4059, #624, #1472, #5078, #11396, #7715, #3382, #7059, #4231, #3152, #4107, #4288, #5135, #8721, #10567, #10679, #504, #6820, #7765, #3210, #6878, #10506, #2309, #680, #4353, #7117, #10742, #2549, #6215, #11639, #3445, #1585, #5253, #8900, #8004, #9267, #11117, #1186, #1059, #10287, #10166, #11172, #4661, #4786, #1962, #3887, #11058, #11235, #5630, #10348, #3046, #2145, #9452, #9392, #10403, #7549, #6596, #1119, #280, #2203 ),
 ( #4725, #2987, #1002, #6716, #2080, #6775, #3829, #5815, #5870, #3110, #3943, #7494, #5692, #4908, #6653, #2929, #10225, #2867, #8500, #5755, #340, #4851, #7606, #8378, #1238, #224, #6534, #8443, #8314, #2018, #8559, #95, #158, #7665, #4005, #11300, #3763, #7431, #9330, #3394, #10457, #634, #10627, #8855, #3163, #5143, #4969, #2376, #11410, #8621, #1483, #9572, #8733, #7778, #2504, #461, #6888, #4241, #5995, #574, #3335, #9686, #9511, #3220, #4296, #7955, #8795, #1302, #403, #11589, #10516, #7068, #4068, #7725, #7900, #10692, #11355, #6833, #5205, #6107, #2259, #4179, #6949, #1369, #8678, #5930, #5032, #4117, #11529, #2323, #9629, #1424, #5087, #516, #7839, #11468, #1538, #3279, #10575, #6051, #7005, #2441, #9740, #5378, #4422, #10979, #8972, #3513, #860, #2616, #9082, #11824, #6343, #6169, #8079, #9139, #921, #1769, #9800, #1594, #4589, #11713, #8245, #690 ),
 ( #5490, #3573, #7243, #22, #3690, #8128, #4532, #2559, #7354, #4362, #747, #10806, #8909, #5262, #8014, #8187, #7182, #11652, #3630, #3461, #5319, #6285, #10750, #10866, #7128, #9916, #6398, #11765, #6226, #1713, #4476, #2678, #9030, #9857, #9974, #1650, #806, #5434, #7299, #10929, #2739, #1820, #10028, #872, #220, #8434, #1056, #6528, #5626, #5686, #3642, #1894, #10877, #4720, #8310, #4780, #1833, #8374, #3883, #1116, #10160, #5503, #3700, #2925, #9209, #9150, #934, #4544, #1957, #4657, #10221, #7426, #9263, #2749, #154, #10096, #9092, #10989, #2688, #4599, #7489, #6354, #6407, #9326, #91, #998, #9983, #2013, #8256, #1778, #11833, #5445, #3820, #8199, #7310, #11111, #10939, #3757, #32, #5563, #10039, #7364, #6591, #11052, #2803, #2860, #6467, #2254, #4846, #10398, #3158, #4964, #5084, #1179, #5029, #1362, #457, #2076, #10513, #8497, #276, #511, #336, #6773 ) ),
 .UNSPECIFIED., .F., .F., .F.,
 ( 4, 4 ),
 ( 4, 2, 2, 2, 2, 2, 2, 2, 2, 2, 2, 2, 2, 2, 2, 2, 2, 2, 2, 2, 2, 2, 2, 2, 2, 2, 2, 2, 2, 2, 2, 2, 2, 2, 2, 2, 2, 2, 2, 2, 2, 2, 2, 2, 2, 2, 2, 2, 2, 2, 2, 2, 2, 2, 2, 2, 2, 2, 2, 2, 2, 4 ),
 ( 0.000000000000000000, 1.000000000000000000 ),
 ( 0.000000000000000000, 0.02499977550252127645, 0.04999988577693819519, 0.07499999605135511394, 0.09999999831535408279, 0.1250000005793530378, 0.1500000028441162425, 0.1750000051088794195, 0.1937500039558066045, 0.2031250033792701970, 0.2125000028027338173, 0.2218750022261974375, 0.2312500016496610300, 0.2500000004965882150, 0.2750000027613288545, 0.3000000050260694384, 0.3187500038730080032, 0.3281250032964772578, 0.3375000027199465125, 0.3468750021434158226, 0.3562500015668850772, 0.3750000004138236420, 0.4000000026785641705, 0.4250000049433046989, 0.4437500037902432082, 0.4531250032137125183, 0.4625000026371817730, 0.4718750020606510276, 0.4812500014841203377, 0.5000000003310588470, 0.5250000025957997085, 0.5500000048605405700, 0.5687500037074788573, 0.5781250031309480564, 0.5875000025544172555, 0.5968750019778864546, 0.6062500014013556537, 0.6250000002482940520, 0.6500000025128280789, 0.6750000047773621059, 0.6937500036244039769, 0.7031250030479249125, 0.7125000024714458480, 0.7218750018949667835, 0.7312500013184877190, 0.7500000001655295900, 0.7750000023794885173, 0.8000000045934475557, 0.8187500034657768655, 0.8281250029019414649, 0.8375000023381060643, 0.8468750017742707747, 0.8562500012104353742, 0.8750000000827646840, 0.8937502654913498379, 0.9031253981956424148, 0.9125005308999349918, 0.9218756636042275687, 0.9312507963085201457, 0.9500010617171052996, 0.9750005308585526498, 1.000000000000000000 ),
 .UNSPECIFIED. ) ;
#5006=CARTESIAN_POINT ( 'NONE',  ( -58.05785365788000263, 64.93276152744238061, 18.60033633024681521 ) ) ;
#5018=CARTESIAN_POINT ( 'NONE',  ( -31.26269038945179446, 34.87416470039633509, 6.107602927758665423 ) ) ;
#5019=ORIENTED_EDGE ( 'NONE', *, *, #7133, .T. ) ;
#5021=CARTESIAN_POINT ( 'NONE',  ( 2.670522128595300249, 35.57712497142318142, -8.044658458458092909 ) ) ;
#5022=CARTESIAN_POINT ( 'NONE',  ( -19.33520177743824320, 64.91269256302088309, 9.913189658205579846 ) ) ;
#5029=CARTESIAN_POINT ( 'NONE',  ( -63.75812180237208793, 55.00413150893107428, -0.006526425526955113854 ) ) ;
#5030=CYLINDRICAL_SURFACE ( 'NONE', #2663, 4.999999999999997335 ) ;
#5032=CARTESIAN_POINT ( 'NONE',  ( -44.75046787418907712, 57.03233382151384490, -6.700212328598206035 ) ) ;
#5034=CARTESIAN_POINT ( 'NONE',  ( -16.69731055678936826, 70.57278980777935828, 14.11442052818484783 ) ) ;
#5036=CARTESIAN_POINT ( 'NONE',  ( 52.99999999999999289, 58.53553390593273065, 3.535533905932731091 ) ) ;
#5040=ORIENTED_EDGE ( 'NONE', *, *, #10185, .T. ) ;
#5045=CARTESIAN_POINT ( 'NONE',  ( -27.49360061100878738, 37.45598436699922473, 11.71495266747331421 ) ) ;
#5046=DIRECTION ( 'NONE',  ( 0.000000000000000000, 1.000000000000000000, 0.000000000000000000 ) ) ;
#5047=PLANE ( 'NONE',  #5690 ) ;
#5053=CARTESIAN_POINT ( 'NONE',  ( -44.65600760483433618, 56.29883701348843772, -4.839347163649881267 ) ) ;
#5056=CARTESIAN_POINT ( 'NONE',  ( -60.66697644449794780, 52.31984451244050405, 6.470678962653597210 ) ) ;
#5058=DIRECTION ( 'NONE',  ( -1.000000000000000000, -0.000000000000000000, -0.000000000000000000 ) ) ;
#5069=CARTESIAN_POINT ( 'NONE',  ( -4.331185467099802899, 55.00135650712124402, -0.002828848648976476851 ) ) ;
#5074=CARTESIAN_POINT ( 'NONE',  ( -44.96936008568403764, 63.99178041037959019, -19.01235157881157178 ) ) ;
#5077=CARTESIAN_POINT ( 'NONE',  ( 15.14427135698260507, 57.74566953878471054, 20.97954867241053023 ) ) ;
#5078=CARTESIAN_POINT ( 'NONE',  ( -31.58948382711383118, 41.58084601413256820, 4.072244092560330486 ) ) ;
#5081=CARTESIAN_POINT ( 'NONE',  ( -25.98930196984718322, 53.70295539467162627, 4.839812903858289772 ) ) ;
#5084=CARTESIAN_POINT ( 'NONE',  ( -62.87201990682712704, 55.00012644727732436, 0.002206787302671962998 ) ) ;
#5087=CARTESIAN_POINT ( 'NONE',  ( -49.22341880855515939, 61.10062350524368924, -3.518778999107284200 ) ) ;
#5089=CARTESIAN_POINT ( 'NONE',  ( -48.85567157503042779, 75.97628680226326026, -2.745941867523475466 ) ) ;
#5096=PRODUCT_DEFINITION_FORMATION_WITH_SPECIFIED_SOURCE ( 'ANY', '', #10824, .NOT_KNOWN. ) ;
#5102=CARTESIAN_POINT ( 'NONE',  ( -22.47759590436300314, 52.25445647903773505, 21.02373912143526979 ) ) ;
#5114=CARTESIAN_POINT ( 'NONE',  ( -52.79191841873938529, 60.62555712573470856, 4.171026843566116860 ) ) ;
#5126=CARTESIAN_POINT ( 'NONE',  ( -17.46186840051235123, 54.99807057725060133, -0.005246742405310452287 ) ) ;
#5132=CARTESIAN_POINT ( 'NONE',  ( -21.32947787934852357, 63.04568470447853912, 19.42265540296757464 ) ) ;
#5134=CARTESIAN_POINT ( 'NONE',  ( -9.302693722564239209, 70.58343099003624843, -14.12448736900078572 ) ) ;
#5135=CARTESIAN_POINT ( 'NONE',  ( -37.20624055104932637, 43.81852209390767428, -8.592061044857116414 ) ) ;
#5142=CARTESIAN_POINT ( 'NONE',  ( 12.14951178748830785, 51.69754629963415482, 3.768454028063179972 ) ) ;
#5143=CARTESIAN_POINT ( 'NONE',  ( -15.77658089785693996, 62.01719014345248837, 0.9163230061594601628 ) ) ;
#5145=CARTESIAN_POINT ( 'NONE',  ( -15.27494751580540111, 73.62981360231496808, 9.945832149094092856 ) ) ;
#5147=CARTESIAN_POINT ( 'NONE',  ( -70.34104699118842063, 33.99562393659818582, 0.006612473344882202446 ) ) ;
#5156=CARTESIAN_POINT ( 'NONE',  ( -17.00387655282055377, 69.86881140706658755, 14.86941770366936311 ) ) ;
#5166=ORIENTED_EDGE ( 'NONE', *, *, #365, .F. ) ;
#5167=DIRECTION ( 'NONE',  ( 0.000000000000000000, 0.000000000000000000, -1.000000000000000000 ) ) ;
#5170=CARTESIAN_POINT ( 'NONE',  ( -39.66652693873400182, 55.00025670080164275, -7.011456267774554441 ) ) ;
#5173=CARTESIAN_POINT ( 'NONE',  ( 47.00000000000000000, 50.00000000000000000, 0.000000000000000000 ) ) ;
#5180=AXIS2_PLACEMENT_3D ( 'NONE', #1992, #10131, #8289 ) ;
#5182=CARTESIAN_POINT ( 'NONE',  ( 6.461783816738637221, 54.99547691306821662, -0.0002561227516112092638 ) ) ;
#5190=CARTESIAN_POINT ( 'NONE',  ( -27.52231952827322559, 42.10572610250680015, 16.77759997522909785 ) ) ;
#5191=ORIENTED_EDGE ( 'NONE', *, *, #9736, .F. ) ;
#5192=CARTESIAN_POINT ( 'NONE',  ( -20.07074684291900368, 64.90603024148451539, 18.53632013344132545 ) ) ;
#5193=CARTESIAN_POINT ( 'NONE',  ( -21.66480673580358385, 60.36362435138872229, 12.94784811284827519 ) ) ;
#5200=EDGE_CURVE ( 'NONE', #3047, #7152, #6636, .T. ) ;
#5203=CARTESIAN_POINT ( 'NONE',  ( 16.81209710897601894, 55.32596159299130534, 5.000262235126429644 ) ) ;
#5205=CARTESIAN_POINT ( 'NONE',  ( -39.89001230141098375, 51.48114101346921245, -6.100591306325558349 ) ) ;
#5207=CARTESIAN_POINT ( 'NONE',  ( 7.391719151893840767, 34.79510180625957361, 6.140032301524222191 ) ) ;
#5209=ADVANCED_FACE ( 'NONE', ( #5673, #2969 ), #262, .F. ) ;
#5217=ADVANCED_FACE ( 'NONE', ( #7532 ), #9741, .T. ) ;
#5218=CARTESIAN_POINT ( 'NONE',  ( -19.63602748969081446, 62.08618401115764129, 19.80343740535094099 ) ) ;
#5222=CARTESIAN_POINT ( 'NONE',  ( -66.03853052622707764, 51.69700120711628699, 3.767903919035947347 ) ) ;
#5225=CARTESIAN_POINT ( 'NONE',  ( -30.67054324275970600, 35.57292846186890500, 8.046485333435041909 ) ) ;
#5230=EDGE_CURVE ( 'NONE', #8109, #7013, #3204, .T. ) ;
#5233=CARTESIAN_POINT ( 'NONE',  ( -30.62461364447335299, 47.99170624137034480, -0.3444639498507808262 ) ) ;
#5243=FACE_OUTER_BOUND ( 'NONE', #8962, .T. ) ;
#5244=CARTESIAN_POINT ( 'NONE',  ( -12.90719201245152270, 54.97644505888057154, -0.01153927764518185815 ) ) ;
#5250=CARTESIAN_POINT ( 'NONE',  ( -56.32961277634869646, 69.86611656190129338, 14.86520567151240080 ) ) ;
#5252=CARTESIAN_POINT ( 'NONE',  ( -55.96940532477286467, 69.12455838185616130, 15.58340920153898956 ) ) ;
#5253=CARTESIAN_POINT ( 'NONE',  ( -53.16357022681673783, 68.79221833313241063, 2.747526514237220052 ) ) ;
#5261=CARTESIAN_POINT ( 'NONE',  ( 24.97984200873575489, 59.96742995076570537, 0.6563446142137170369 ) ) ;
#5262=CARTESIAN_POINT ( 'NONE',  ( 7.240609414712229963, 54.98725137911733896, 0.01040343736786853227 ) ) ;
#5263=ORIENTED_EDGE ( 'NONE', *, *, #11755, .T. ) ;
#5264=CARTESIAN_POINT ( 'NONE',  ( -8.636027272868737725, 70.58382813124079291, -14.12485756978424334 ) ) ;
#5273=CARTESIAN_POINT ( 'NONE',  ( -40.03064391692543467, 53.96877717286832876, -20.99202776130344361 ) ) ;
#5285=CARTESIAN_POINT ( 'NONE',  ( -59.20813656377777079, 53.97164354997492808, 6.936260356707947494 ) ) ;
#5300=CARTESIAN_POINT ( 'NONE',  ( -17.75699671169975957, 54.99635662262475222, -0.009584463525143764942 ) ) ;
#5304=EDGE_LOOP ( 'NONE', ( #4511, #10915 ) ) ;
#5308=CARTESIAN_POINT ( 'NONE',  ( -57.39118702654079129, 64.93227794977589440, 18.59917511543459767 ) ) ;
#5311=CIRCLE ( 'NONE', #4150, 9.999999999999987566 ) ;
#5314=CARTESIAN_POINT ( 'NONE',  ( 24.18742635297404675, 76.02379904146428657, 2.751050496637376774 ) ) ;
#5319=CARTESIAN_POINT ( 'NONE',  ( 2.461783834978326091, 54.99737575019351254, -0.0002517746684140311744 ) ) ;
#5321=CARTESIAN_POINT ( 'NONE',  ( -13.81096152673235800, 76.02210280262706021, 2.745652712408400031 ) ) ;
#5322=CARTESIAN_POINT ( 'NONE',  ( 2.003855453843550460, 35.57695044197526357, -8.044733130177707636 ) ) ;
#5330=CARTESIAN_POINT ( 'NONE',  ( -63.67978690865925984, 51.02815575133915615, 3.054710809982001507 ) ) ;
#5332=CARTESIAN_POINT ( 'NONE',  ( -61.63584152524990145, 46.00569487729882212, 19.01260273971552905 ) ) ;
#5336=CARTESIAN_POINT ( 'NONE',  ( -56.32252171033144350, 58.97418346094907804, 3.051949254714778625 ) ) ;
#5339=CARTESIAN_POINT ( 'NONE',  ( 6.681748455246894203, 50.66235202709670915, 2.508378333353272982 ) ) ;
#5346=CARTESIAN_POINT ( 'NONE',  ( -3.016088031971444039, 55.65411387417407951, -4.967671222318850610 ) ) ;
#5348=CARTESIAN_POINT ( 'NONE',  ( -13.53949924236008862, 68.61239594966130539, 3.656398761500181838 ) ) ;
#5359=CARTESIAN_POINT ( 'NONE',  ( -28.24307224120747861, 54.99071020490737993, 0.002851684764032580855 ) ) ;
#5364=CARTESIAN_POINT ( 'NONE',  ( -22.84604256752122708, 53.39459927986023757, 4.746710467859072580 ) ) ;
#5365=CARTESIAN_POINT ( 'NONE',  ( -54.88146047731135013, 73.03677976846768161, 10.81065700633557825 ) ) ;
#5367=CARTESIAN_POINT ( 'NONE',  ( -43.40408007066994145, 61.10253656447230952, -20.11177873753167589 ) ) ;
#5372=CARTESIAN_POINT ( 'NONE',  ( 17.18896242946999919, 60.50854855881860317, 20.47421955154796436 ) ) ;
#5378=CARTESIAN_POINT ( 'NONE',  ( -57.00013066340230949, 59.95461989290591731, 4.954166194309457261 ) ) ;
#5379=EDGE_LOOP ( 'NONE', ( #7275, #5166, #6073, #4764 ) ) ;
#5380=CARTESIAN_POINT ( 'NONE',  ( -2.144294859876037851, 49.49184188862220424, -20.47260631371810291 ) ) ;
#5381=VECTOR ( 'NONE', #6912, 1000.000000000000000 ) ;
#5383=CARTESIAN_POINT ( 'NONE',  ( -41.16026710375170694, 50.89060761561553647, -20.69263693287480521 ) ) ;
#5394=VECTOR ( 'NONE', #4982, 1000.000000000000000 ) ;
#5396=ORIENTED_EDGE ( 'NONE', *, *, #9953, .T. ) ;
#5397=CYLINDRICAL_SURFACE ( 'NONE', #5515, 9.999999999999987566 ) ;
#5402=EDGE_LOOP ( 'NONE', ( #6319, #10792 ) ) ;
#5405=CARTESIAN_POINT ( 'NONE',  ( 3.983988775803998905, 50.66121500187745852, -2.506212315349996445 ) ) ;
#5406=CARTESIAN_POINT ( 'NONE',  ( 10.53956211717208014, 43.78843572598016465, 8.622155805075909285 ) ) ;
#5408=EDGE_CURVE ( 'NONE', #3592, #1675, #7656, .T. ) ;
#5417=CARTESIAN_POINT ( 'NONE',  ( -50.99787495343821320, 55.00280540214748726, 0.001329527542247992220 ) ) ;
#5421=ORIENTED_EDGE ( 'NONE', *, *, #3201, .F. ) ;
#5422=CARTESIAN_POINT ( 'NONE',  ( -61.88037028687247698, 51.91449295574040690, 20.80032498971814192 ) ) ;
#5424=CARTESIAN_POINT ( 'NONE',  ( -60.33823637602682766, 55.00059828005016982, 21.02834956124393884 ) ) ;
#5429=CARTESIAN_POINT ( 'NONE',  ( -11.52239577449127061, 75.97627689174807131, -2.745668057393931161 ) ) ;
#5434=CARTESIAN_POINT ( 'NONE',  ( -9.795201718507710709, 54.99722681578106886, 0.002449751363073274148 ) ) ;
#5436=ADVANCED_FACE ( 'NONE', ( #7138 ), #11724, .F. ) ;
#5437=CARTESIAN_POINT ( 'NONE',  ( 4.785240962488377825, 34.19851723175345626, -3.085388102356358075 ) ) ;
#5438=CARTESIAN_POINT ( 'NONE',  ( -42.33720994522852266, 55.00043528610386545, -21.02753041772728437 ) ) ;
#5445=CARTESIAN_POINT ( 'NONE',  ( -48.75936011024216299, 55.01274827867656114, -0.01040309443492500041 ) ) ;
#5446=CARTESIAN_POINT ( 'NONE',  ( -33.35108528763237956, 50.66059424145658596, -2.505263451482964143 ) ) ;
#5449=CARTESIAN_POINT ( 'NONE',  ( -70.70219505483254352, 49.99995498154407159, 0.3302917765627791380 ) ) ;
#5461=CARTESIAN_POINT ( 'NONE',  ( -10.46040627582160099, 68.65766219505340473, -3.675420389180045433 ) ) ;
#5464=MECHANICAL_DESIGN_GEOMETRIC_PRESENTATION_REPRESENTATION('',(#4316),#11372);
#5471=CARTESIAN_POINT ( 'NONE',  ( -42.82983869248258912, 55.00187443791501352, -0.004031347153255517880 ) ) ;
#5474=CARTESIAN_POINT ( 'NONE',  ( -8.852116072238684907, 59.49383071322154848, -2.216568777849228677 ) ) ;
#5478=ORIENTED_EDGE ( 'NONE', *, *, #899, .T. ) ;
#5479=CARTESIAN_POINT ( 'NONE',  ( 3.451907635234679361, 34.19915017745972108, -3.085386652995293133 ) ) ;
#5485=CARTESIAN_POINT ( 'NONE',  ( -17.59602449223222109, 68.34579465778965357, 16.25793134507749826 ) ) ;
#5490=CARTESIAN_POINT ( 'NONE',  ( 22.00000000000000711, 54.99999999999999289, 0.000000000000000000 ) ) ;
#5492=CARTESIAN_POINT ( 'NONE',  ( -35.52239577659344860, 38.22489504150217243, -12.89214396572665500 ) ) ;
#5493=VECTOR ( 'NONE', #1482, 1000.000000000000000 ) ;
#5494=CARTESIAN_POINT ( 'NONE',  ( 0.8268573817076104726, 37.44832105976551873, -11.71822709476406210 ) ) ;
#5503=CARTESIAN_POINT ( 'NONE',  ( -27.75939058475275800, 54.99220303251508568, 0.01449020901263564122 ) ) ;
#5504=CARTESIAN_POINT ( 'NONE',  ( -52.01616715382184708, 59.33866825769318609, 2.506581953018356845 ) ) ;
#5510=CARTESIAN_POINT ( 'NONE',  ( -8.839809468419982608, 72.54364378520992318, -11.73195350307014273 ) ) ;
#5512=CARTESIAN_POINT ( 'NONE',  ( 20.68040016808398107, 59.84041032842515762, 1.294695803031751247 ) ) ;
#5515=AXIS2_PLACEMENT_3D ( 'NONE', #7086, #8204, #10887 ) ;
#5520=CARTESIAN_POINT ( 'NONE',  ( -5.589484852938766402, 61.61028781279477329, -12.37056010730757194 ) ) ;
#5524=ORIENTED_EDGE ( 'NONE', *, *, #11792, .F. ) ;
#5530=CARTESIAN_POINT ( 'NONE',  ( -66.57380018018302792, 55.02491533713232030, -0.005784342931633022940 ) ) ;
#5534=CARTESIAN_POINT ( 'NONE',  ( -21.68459333372202735, 54.34592763142354244, 4.967663218408093329 ) ) ;
#5539=CARTESIAN_POINT ( 'NONE',  ( 19.85574934264614910, 73.36821619702706698, 10.58005382006121131 ) ) ;
#5547=CARTESIAN_POINT ( 'NONE',  ( -39.16026728571524984, 50.89059911655681390, -20.69167526169209026 ) ) ;
#5548=CARTESIAN_POINT ( 'NONE',  ( -41.21475901749523274, 58.08538884819615333, -20.80179922188357011 ) ) ;
#5551=CARTESIAN_POINT ( 'NONE',  ( 62.44550000000000267, 55.00000000000000000, 0.000000000000000000 ) ) ;
#5555=CARTESIAN_POINT ( 'NONE',  ( -49.52233824455085909, 75.97792204488571599, -2.745941792655960167 ) ) ;
#5556=CARTESIAN_POINT ( 'NONE',  ( -26.81096152405270061, 44.41979049410412017, 18.36814973051028588 ) ) ;
#5561=ORIENTED_EDGE ( 'NONE', *, *, #7905, .T. ) ;
#5563=CARTESIAN_POINT ( 'NONE',  ( -55.57639901084645828, 55.00517665877310236, 0.003022361695382154087 ) ) ;
#5564=CARTESIAN_POINT ( 'NONE',  ( -61.34696192836374706, 52.49897595166400777, 4.332661177462228785 ) ) ;
#5566=DIRECTION ( 'NONE',  ( 1.000000000000000000, 6.033820786006286457E-17, -0.000000000000000000 ) ) ;
#5569=CARTESIAN_POINT ( 'NONE',  ( 19.52230480204648799, 67.92440004991483704, 16.80766691833610693 ) ) ;
#5573=CARTESIAN_POINT ( 'NONE',  ( 5.513839465024632069, 50.25394865510380527, 1.607139511838376000 ) ) ;
#5580=FACE_OUTER_BOUND ( 'NONE', #5402, .T. ) ;
#5581=AXIS2_PLACEMENT_3D ( 'NONE', #1791, #10178, #9163 ) ;
#5583=CARTESIAN_POINT ( 'NONE',  ( -19.29698723374914593, 59.72494936439868951, 13.20503860676303098 ) ) ;
#5599=CARTESIAN_POINT ( 'NONE',  ( -65.75702278283388580, 54.97107188852366733, 0.01144463408162874063 ) ) ;
#5604=DIRECTION ( 'NONE',  ( 1.000000000000000000, 6.033820786006286457E-17, -0.000000000000000000 ) ) ;
#5607=CARTESIAN_POINT ( 'NONE',  ( 6.058385820703728442, 34.79737119409461599, 6.139092558150637480 ) ) ;
#5610=CARTESIAN_POINT ( 'NONE',  ( -13.85565285731654761, 75.43037139504293975, 5.490367781071763709 ) ) ;
#5611=( LENGTH_UNIT ( ) NAMED_UNIT ( * ) SI_UNIT ( .MILLI., .METRE. ) );
#5612=CARTESIAN_POINT ( 'NONE',  ( -52.00383529082647271, 74.42722782460430153, 8.047526119559261559 ) ) ;
#5615=CARTESIAN_POINT ( 'NONE',  ( 3.571755578639977724, 50.00000000000001421, 2.874253840576960811E-12 ) ) ;
#5618=CARTESIAN_POINT ( 'NONE',  ( -21.17314274085600090, 59.12512438474372090, 20.69754144995899026 ) ) ;
#5619=CARTESIAN_POINT ( 'NONE',  ( -59.27472368810988002, 61.13901599248961105, 20.20251803659174783 ) ) ;
#5626=CARTESIAN_POINT ( 'NONE',  ( -18.83686826543840453, 54.99741186838863882, -0.002939892491207554172 ) ) ;
#5627=CARTESIAN_POINT ( 'NONE',  ( -49.68512622689396352, 59.96742314939218943, 0.6560827949113757773 ) ) ;
#5630=CARTESIAN_POINT ( 'NONE',  ( -62.21092016019122894, 52.94303745291883700, 13.86761892224957116 ) ) ;
#5634=VECTOR ( 'NONE', #8505, 1000.000000000000000 ) ;
#5643=CARTESIAN_POINT ( 'NONE',  ( -32.40470529452398551, 41.55719028461663100, -4.081861330394077392 ) ) ;
#5647=VERTEX_POINT ( 'NONE', #8981 ) ;
#5653=CARTESIAN_POINT ( 'NONE',  ( -14.58248992847019920, 61.22172256553918146, 3.321057901781169885 ) ) ;
#5655=VECTOR ( 'NONE', #8671, 1000.000000000000000 ) ;
#5659=DIRECTION ( 'NONE',  ( 0.000000000000000000, 0.000000000000000000, 1.000000000000000000 ) ) ;
#5664=CARTESIAN_POINT ( 'NONE',  ( -1.144262565995328940, 42.07883645215377300, -16.80394782698530065 ) ) ;
#5669=CARTESIAN_POINT ( 'NONE',  ( -2.188986190505546769, 52.25407376895000056, -20.97627476078892528 ) ) ;
#5670=CARTESIAN_POINT ( 'NONE',  ( -34.14426257084027583, 36.62727174719971401, -10.58198811264723282 ) ) ;
#5673=FACE_BOUND ( 'NONE', #7111, .T. ) ;
#5674=CARTESIAN_POINT ( 'NONE',  ( 19.85574934264614910, 73.36821619702706698, 10.58005382006121131 ) ) ;
#5677=CARTESIAN_POINT ( 'NONE',  ( -15.94161418140128994, 73.62867900310379810, 9.945362048789077036 ) ) ;
#5678=CARTESIAN_POINT ( 'NONE',  ( 10.20626039314592681, 47.94399561767391305, 12.25029052866368673 ) ) ;
#5684=EDGE_LOOP ( 'NONE', ( #7095, #10828, #11669, #5524 ) ) ;
#5686=CARTESIAN_POINT ( 'NONE',  ( -19.71439386582751752, 54.99634062743773910, -0.004164711759880548002 ) ) ;
#5687=CARTESIAN_POINT ( 'NONE',  ( -53.95632792247587162, 58.30500826365688738, 3.766154981294819404 ) ) ;
#5690=AXIS2_PLACEMENT_3D ( 'NONE', #11546, #8694, #6733 ) ;
#5692=CARTESIAN_POINT ( 'NONE',  ( 9.109914677241386372, 50.71033554483514649, 5.585537211039464545 ) ) ;
#5695=CARTESIAN_POINT ( 'NONE',  ( 23.47754340821147068, 75.43020022661498558, 5.490793176664390707 ) ) ;
#5696=DIRECTION ( 'NONE',  ( 1.000000000000000000, 6.033820786006286457E-17, -0.000000000000000000 ) ) ;
#5702=CIRCLE ( 'NONE', #6665, 4.999999999999984013 ) ;
#5707=CARTESIAN_POINT ( 'NONE',  ( -50.49690380378408605, 68.79103478457420806, 2.747024645387534214 ) ) ;
#5716=CARTESIAN_POINT ( 'NONE',  ( 53.00000000000000000, 51.46446609406726935, 3.535533905932731091 ) ) ;
#5718=EDGE_CURVE ( 'NONE', #5990, #443, #3243, .T. ) ;
#5720=CARTESIAN_POINT ( 'NONE',  ( -67.32905043534587719, 54.99390458312336705, -0.002695445133683335107 ) ) ;
#5723=DIRECTION ( 'NONE',  ( 0.000000000000000000, -1.000000000000000000, 0.000000000000000000 ) ) ;
#5728=ORIENTED_EDGE ( 'NONE', *, *, #4409, .T. ) ;
#5729=CARTESIAN_POINT ( 'NONE',  ( -31.26269038945179446, 34.87416470039633509, 6.107602927758665423 ) ) ;
#5731=CARTESIAN_POINT ( 'NONE',  ( -58.69833756168564065, 56.03204939003842355, 20.99267139547387373 ) ) ;
#5737=CARTESIAN_POINT ( 'NONE',  ( 1.627231888947060723, 50.25466374745918330, -1.609084181729487639 ) ) ;
#5738=CARTESIAN_POINT ( 'NONE',  ( 9.810937555461070048, 42.10554236623130464, 16.77741859935663626 ) ) ;
#5740=CARTESIAN_POINT ( 'NONE',  ( -39.82693389173066834, 50.89060194957639283, -20.69199581875299643 ) ) ;
#5741=CARTESIAN_POINT ( 'NONE',  ( -50.85567158358731632, 75.98119253013058483, -2.745941642920928683 ) ) ;
#5751=DIRECTION ( 'NONE',  ( 0.000000000000000000, 1.000000000000000000, 0.000000000000000000 ) ) ;
#5755=CARTESIAN_POINT ( 'NONE',  ( 3.083722735221986255, 48.01900164405483196, -0.6869154824850737251 ) ) ;
#5757=CARTESIAN_POINT ( 'NONE',  ( 4.003855478097921861, 35.57747403031575573, -8.044509115018048107 ) ) ;
#5759=DIRECTION ( 'NONE',  ( 9.813077866773612233E-16, -1.000000000000000000, -0.000000000000000000 ) ) ;
#5767=CARTESIAN_POINT ( 'NONE',  ( -60.40957880102118338, 50.93284021614062596, 13.40225281893947340 ) ) ;
#5774=CIRCLE ( 'NONE', #6546, 4.999999999999997335 ) ;
#5778=CARTESIAN_POINT ( 'NONE',  ( -51.65302243398222970, 59.96738868206218598, -0.6562502162082396451 ) ) ;
#5781=CARTESIAN_POINT ( 'NONE',  ( -5.541508246797579140, 58.60498886477284941, -6.015263639686886599 ) ) ;
#5786=VECTOR ( 'NONE', #4401, 1000.000000000000000 ) ;
#5792=CARTESIAN_POINT ( 'NONE',  ( -48.52239103406665066, 73.33336493528216238, -10.56581381373428208 ) ) ;
#5797=CARTESIAN_POINT ( 'NONE',  ( -78.00000000000000000, 50.00000000000000000, 6.123233995736758394E-16 ) ) ;
#5800=CARTESIAN_POINT ( 'NONE',  ( -0.3234080915047974902, 51.02589827434706393, -3.051885828346310614 ) ) ;
#5802=ORIENTED_EDGE ( 'NONE', *, *, #10537, .F. ) ;
#5803=CARTESIAN_POINT ( 'NONE',  ( 8.144347139672229119, 36.66824632778702409, 10.56543010816455386 ) ) ;
#5804=CARTESIAN_POINT ( 'NONE',  ( -45.83980951013849392, 66.71822699054862937, -17.55167914569291554 ) ) ;
#5812=ADVANCED_FACE ( 'NONE', ( #4957 ), #7828, .F. ) ;
#5815=CARTESIAN_POINT ( 'NONE',  ( 14.55667984625315015, 56.83871188529325025, 6.833734452169164086 ) ) ;
#5817=CARTESIAN_POINT ( 'NONE',  ( -42.07074724807011989, 61.10209548959944215, -20.11061483308460751 ) ) ;
#5824=ORIENTED_EDGE ( 'NONE', *, *, #7193, .T. ) ;
#5828=CARTESIAN_POINT ( 'NONE',  ( -52.54481729858026995, 67.02647195319831042, 7.208015641604088586 ) ) ;
#5835=CARTESIAN_POINT ( 'NONE',  ( -45.04238000299608302, 56.61143717230429928, -4.744501108842417381 ) ) ;
#5837=CARTESIAN_POINT ( 'NONE',  ( -13.22334562740580921, 61.79442050427090294, 1.822429741926403501 ) ) ;
#5839=FACE_OUTER_BOUND ( 'NONE', #10994, .T. ) ;
#5841=CYLINDRICAL_SURFACE ( 'NONE', #8364, 4.999999999999984013 ) ;
#5844=CARTESIAN_POINT ( 'NONE',  ( -55.73751408985167899, 71.24607175163586703, 13.33484869932101269 ) ) ;
#5855=CARTESIAN_POINT ( 'NONE',  ( -33.30269350532120143, 33.99387206627966407, -1.031609878214063025 ) ) ;
#5859=CARTESIAN_POINT ( 'NONE',  ( 23.66666666666668561, 76.00000000000000000, 0.000000000000000000 ) ) ;
#5860=CARTESIAN_POINT ( 'NONE',  ( 18.79384863814433615, 66.18161908153624040, 8.591911950030317158 ) ) ;
#5862=PLANE ( 'NONE',  #7194 ) ;
#5864=EDGE_LOOP ( 'NONE', ( #2588, #3582, #8242, #5191 ) ) ;
#5870=CARTESIAN_POINT ( 'NONE',  ( 13.77658176772798093, 55.91632091561838536, 6.982821974894761752 ) ) ;
#5872=CARTESIAN_POINT ( 'NONE',  ( -43.83980969374544401, 66.71858909844225138, -17.55257377017560216 ) ) ;
#5883=CARTESIAN_POINT ( 'NONE',  ( -29.78863982673286870, 41.14007247853228222, 2.056775689438067989 ) ) ;
#5895=CARTESIAN_POINT ( 'NONE',  ( -42.31849960451753390, 54.34441004806944875, -4.967488205851171124 ) ) ;
#5896=ORIENTED_EDGE ( 'NONE', *, *, #11787, .T. ) ;
#5897=CARTESIAN_POINT ( 'NONE',  ( 10.89008576165924680, 49.38437030094291913, 4.319752267554956227 ) ) ;
#5904=CARTESIAN_POINT ( 'NONE',  ( -38.47762819156672265, 42.07891330237754346, -16.80402559754432801 ) ) ;
#5914=CARTESIAN_POINT ( 'NONE',  ( -36.85572911278101316, 38.22258139949027367, -12.89445763391127464 ) ) ;
#5916=CARTESIAN_POINT ( 'NONE',  ( -16.60828084699550544, 73.62754440388609112, 9.944891948484055888 ) ) ;
#5917=CARTESIAN_POINT ( 'NONE',  ( -9.998140069271334696, 64.90968168482568501, -9.910269716092365400 ) ) ;
#5922=DIRECTION ( 'NONE',  ( 1.000000000000000000, 6.033820786006286457E-17, -0.000000000000000000 ) ) ;
#5927=CARTESIAN_POINT ( 'NONE',  ( 47.00000000000000000, 55.00000000000000000, 0.000000000000000000 ) ) ;
#5929=CARTESIAN_POINT ( 'NONE',  ( 47.00000000000000000, 51.46446609406726935, -3.535533905932738197 ) ) ;
#5930=CARTESIAN_POINT ( 'NONE',  ( -44.45858743606044072, 56.70130388464480831, -6.794919630703683211 ) ) ;
#5933=CARTESIAN_POINT ( 'NONE',  ( -18.45202553953894764, 65.80723110900194683, 18.02933743899848551 ) ) ;
#5940=CARTESIAN_POINT ( 'NONE',  ( 36.99999999999999289, 59.99999999999998579, 0.000000000000000000 ) ) ;
#5948=CARTESIAN_POINT ( 'NONE',  ( -4.160267277967630406, 59.12176995062825569, -20.68921489609442332 ) ) ;
#5949=FACE_OUTER_BOUND ( 'NONE', #1859, .T. ) ;
#5952=CARTESIAN_POINT ( 'NONE',  ( 62.44550000000000267, 55.00000000000000000, -2.999999999999995559 ) ) ;
#5953=EDGE_CURVE ( 'NONE', #678, #3881, #10493, .T. ) ;
#5954=ORIENTED_EDGE ( 'NONE', *, *, #149, .T. ) ;
#5959=CARTESIAN_POINT ( 'NONE',  ( 37.00000000000000000, 60.00000000000000000, 6.123233995736769241E-16 ) ) ;
#5962=CARTESIAN_POINT ( 'NONE',  ( -32.08425350687716104, 48.28742629341236636, -2.036605179622332784 ) ) ;
#5968=EDGE_CURVE ( 'NONE', #1776, #10196, #7685, .T. ) ;
#5980=DIRECTION ( 'NONE',  ( -6.033820786006286457E-17, 1.000000000000000000, 0.000000000000000000 ) ) ;
#5983=CARTESIAN_POINT ( 'NONE',  ( -29.49360042904642043, 37.45509264529403737, 11.71531283165970727 ) ) ;
#5985=CARTESIAN_POINT ( 'NONE',  ( -5.493600489990522640, 59.12202052924457973, -20.68980504072543170 ) ) ;
#5986=CARTESIAN_POINT ( 'NONE',  ( -21.96365303252882839, 59.72418919812645299, 13.20300428545286131 ) ) ;
#5990=VERTEX_POINT ( 'NONE', #5959 ) ;
#5995=CARTESIAN_POINT ( 'NONE',  ( -23.75092017888364282, 55.68721295373460833, 6.987118555467080938 ) ) ;
#5997=CARTESIAN_POINT ( 'NONE',  ( -32.72515708217407138, 34.82695427582095959, -6.127117481167428714 ) ) ;
#5998=CARTESIAN_POINT ( 'NONE',  ( 16.81101720596863203, 65.56606704192360269, 18.33326034385300574 ) ) ;
#6007=LINE ( 'NONE', #6846, #5394 ) ;
#6008=CARTESIAN_POINT ( 'NONE',  ( 5.737308841168996310, 34.06700459503902323, -2.059191599423306318 ) ) ;
#6016=LINE ( 'NONE', #8876, #3631 ) ;
#6019=CARTESIAN_POINT ( 'NONE',  ( -26.83355706786435491, 49.15565477916797477, 3.903659954469548055 ) ) ;
#6030=CARTESIAN_POINT ( 'NONE',  ( 3.571755578639977724, 50.00000000000001421, 2.874253840576960811E-12 ) ) ;
#6031=CARTESIAN_POINT ( 'NONE',  ( -15.71439516195324515, 54.99396298233272518, -0.006381203918883474741 ) ) ;
#6037=CARTESIAN_POINT ( 'NONE',  ( -23.05849041873830885, 57.05917197429855037, 20.98589082339331569 ) ) ;
#6039=CARTESIAN_POINT ( 'NONE',  ( -6.363976791488124007, 62.08095487955036162, -19.78975161862042498 ) ) ;
#6040=CARTESIAN_POINT ( 'NONE',  ( -23.40470529880934691, 56.37319246401821005, 13.98650468942532399 ) ) ;
#6043=CARTESIAN_POINT ( 'NONE',  ( -22.87671376304905735, 56.30254047324378064, 4.871888488731487499 ) ) ;
#6051=CARTESIAN_POINT ( 'NONE',  ( -55.24961050147904729, 61.18673322028157457, 3.306144321554119525 ) ) ;
#6053=CARTESIAN_POINT ( 'NONE',  ( -40.03064391692543467, 53.96877717286832876, -20.99202776130344361 ) ) ;
#6057=EDGE_CURVE ( 'NONE', #7152, #11420, #6016, .T. ) ;
#6058=FACE_OUTER_BOUND ( 'NONE', #7034, .T. ) ;
#6065=CARTESIAN_POINT ( 'NONE',  ( -18.45202553953894764, 65.80723110900194683, 18.02933743899848551 ) ) ;
#6073=ORIENTED_EDGE ( 'NONE', *, *, #4803, .F. ) ;
#6078=CARTESIAN_POINT ( 'NONE',  ( -40.24961187995522494, 55.68701082057744145, -6.984114430637439419 ) ) ;
#6089=CARTESIAN_POINT ( 'NONE',  ( 3.836827854034411178, 54.99596874490445231, -0.001874240170360355487 ) ) ;
#6090=AXIS2_PLACEMENT_3D ( 'NONE', #4067, #11409, #339 ) ;
#6094=CARTESIAN_POINT ( 'NONE',  ( -43.78535878948660098, 60.10716095388539060, -20.39140800440753054 ) ) ;
#6096=CARTESIAN_POINT ( 'NONE',  ( -41.67054327082605880, 55.00043308847957491, -21.02772144221139783 ) ) ;
#6097=CARTESIAN_POINT ( 'NONE',  ( -15.46043787753367305, 69.01800930915912602, 1.830987716616894412 ) ) ;
#6104=CARTESIAN_POINT ( 'NONE',  ( 9.477680475861957277, 36.67126955513442255, 10.56417786655960356 ) ) ;
#6106=CARTESIAN_POINT ( 'NONE',  ( 7.095683716263478047, 50.00000000000005684, 2.757939276259992832E-15 ) ) ;
#6107=CARTESIAN_POINT ( 'NONE',  ( -41.24915659003143276, 52.95126970601198479, -6.742091308054726895 ) ) ;
#6109=EDGE_CURVE ( 'NONE', #11411, #10886, #3066, .T. ) ;
#6110=CARTESIAN_POINT ( 'NONE',  ( 14.18903896197797287, 52.25434875799748369, 21.02210295667673989 ) ) ;
#6119=CARTESIAN_POINT ( 'NONE',  ( 4.595919313165082620, 34.88938507153989832, -6.102095433906166377 ) ) ;
#6126=CARTESIAN_POINT ( 'NONE',  ( -31.54809236465146682, 34.60179423563022283, 5.109615027512485419 ) ) ;
#6132=DIRECTION ( 'NONE',  ( 0.000000000000000000, 0.000000000000000000, 1.000000000000000000 ) ) ;
#6134=CARTESIAN_POINT ( 'NONE',  ( -56.58242889277405396, 57.05108172246632137, 6.747627424565906473 ) ) ;
#6143=EDGE_CURVE ( 'NONE', #7749, #1776, #2726, .T. ) ;
#6147=CARTESIAN_POINT ( 'NONE',  ( -7.829838812692313077, 55.00327426656686214, -0.003007153403177842931 ) ) ;
#6153=CARTESIAN_POINT ( 'NONE',  ( -60.69833702282029009, 56.03208645306531110, 20.99415308669729541 ) ) ;
#6155=CARTESIAN_POINT ( 'NONE',  ( -26.14429485881147741, 44.41916384679638696, 18.36966221812192401 ) ) ;
#6156=EDGE_CURVE ( 'NONE', #2139, #5990, #712, .T. ) ;
#6157=CARTESIAN_POINT ( 'NONE',  ( -29.26205205118023400, 44.11983436432798555, 8.937929964154781359 ) ) ;
#6163=CARTESIAN_POINT ( 'NONE',  ( 21.14436220910852882, 71.77416011014268804, 12.89076390558360075 ) ) ;
#6164=CARTESIAN_POINT ( 'NONE',  ( 0.000000000000000000, 0.000000000000000000, 0.000000000000000000 ) ) ;
#6165=ORIENTED_EDGE ( 'NONE', *, *, #3095, .F. ) ;
#6168=CARTESIAN_POINT ( 'NONE',  ( 17.98255850431752378, 56.29716720365202320, 4.839784152412198281 ) ) ;
#6169=CARTESIAN_POINT ( 'NONE',  ( -63.12525701739682660, 53.29900530425329208, 6.794067530835293134 ) ) ;
#6171=CARTESIAN_POINT ( 'NONE',  ( -64.47562408583945626, 38.19583575827792288, 12.92744520505189953 ) ) ;
#6178=EDGE_LOOP ( 'NONE', ( #9023, #10136 ) ) ;
#6181=CARTESIAN_POINT ( 'NONE',  ( -64.46266331143226580, 50.66432291203608429, 2.511714366154293110 ) ) ;
#6182=CARTESIAN_POINT ( 'NONE',  ( -48.85567157503042779, 75.97628680226326026, -2.745941867523475466 ) ) ;
#6187=CARTESIAN_POINT ( 'NONE',  ( -64.86454813115628326, 52.49943474288868828, 4.342307377127885282 ) ) ;
#6190=CARTESIAN_POINT ( 'NONE',  ( 9.009704903381607011, 51.94883714271350783, 3.974653465714529155 ) ) ;
#6193=CARTESIAN_POINT ( 'NONE',  ( 47.00000000000000000, 60.00000000000000000, 6.123233995736766282E-16 ) ) ;
#6197=CARTESIAN_POINT ( 'NONE',  ( -43.16649569290354549, 58.90744599142516336, -5.853545488159599408 ) ) ;
#6206=DIRECTION ( 'NONE',  ( 0.000000000000000000, 1.000000000000000000, 0.000000000000000000 ) ) ;
#6207=CARTESIAN_POINT ( 'NONE',  ( -2.569594468081864314, 55.00124604138196815, -0.01964962527651127611 ) ) ;
#6210=CARTESIAN_POINT ( 'NONE',  ( -14.28778386244584730, 59.49503363445350601, 2.214355864345136649 ) ) ;
#6211=AXIS2_PLACEMENT_3D ( 'NONE', #9034, #11106, #927 ) ;
#6214=CARTESIAN_POINT ( 'NONE',  ( -39.94161417541742054, 48.86043757236269158, -20.20376349713652075 ) ) ;
#6215=CARTESIAN_POINT ( 'NONE',  ( -48.87290492130438935, 67.21699422026077286, -7.042296406420784471 ) ) ;
#6226=CARTESIAN_POINT ( 'NONE',  ( -2.907263427868458816, 55.00473918814381591, 0.01574419816156069629 ) ) ;
#6228=CARTESIAN_POINT ( 'NONE',  ( 11.14427089164646212, 42.10785603453369674, 16.77510495723129580 ) ) ;
#6229=CARTESIAN_POINT ( 'NONE',  ( -1.144262565995328940, 42.07883645215377300, -16.80394782698530065 ) ) ;
#6239=VECTOR ( 'NONE', #6706, 1000.000000000000000 ) ;
#6240=CARTESIAN_POINT ( 'NONE',  ( -40.92935782463053584, 57.05919160630219977, -20.93299540428984429 ) ) ;
#6243=CARTESIAN_POINT ( 'NONE',  ( -52.81739729106450909, 59.99999999999995737, 0.3296920225250882797 ) ) ;
#6248=CARTESIAN_POINT ( 'NONE',  ( 9.791712712594932810, 52.49391147245050604, 4.339007403345378933 ) ) ;
#6254=CARTESIAN_POINT ( 'NONE',  ( -3.791298217890237687, 56.29168220040835280, -4.841196073966652413 ) ) ;
#6255=EDGE_CURVE ( 'NONE', #1817, #1114, #9877, .T. ) ;
#6256=CARTESIAN_POINT ( 'NONE',  ( -4.703005425211010504, 59.71918865705544732, -13.18981795474766194 ) ) ;
#6262=ORIENTED_EDGE ( 'NONE', *, *, #3608, .T. ) ;
#6267=CARTESIAN_POINT ( 'NONE',  ( -41.09033010249994788, 54.99579895668967566, 0.009353565326378111486 ) ) ;
#6274=CARTESIAN_POINT ( 'NONE',  ( -56.63607177307330431, 69.12418599258134577, 15.58301102096070245 ) ) ;
#6276=CARTESIAN_POINT ( 'NONE',  ( -53.03060745306661516, 74.78972051499107465, 7.080976978603892746 ) ) ;
#6281=LINE ( 'NONE', #9025, #2016 ) ;
#6284=CARTESIAN_POINT ( 'NONE',  ( 17.20429921762959324, 55.65812106999769782, 4.967195391103087942 ) ) ;
#6285=CARTESIAN_POINT ( 'NONE',  ( 1.871464948240592063, 55.00332452672969907, 0.001624608827728054976 ) ) ;
#6287=CARTESIAN_POINT ( 'NONE',  ( -0.5223957761089466079, 44.43543377721479004, -18.33034268388519195 ) ) ;
#6288=CARTESIAN_POINT ( 'NONE',  ( -17.27494751259140315, 73.62640980466187557, 9.944421848179040069 ) ) ;
#6295=DIRECTION ( 'NONE',  ( 0.000000000000000000, -0.000000000000000000, 1.000000000000000000 ) ) ;
#6303=FACE_OUTER_BOUND ( 'NONE', #2617, .T. ) ;
#6304=CARTESIAN_POINT ( 'NONE',  ( -70.34104699118840642, 33.99562393659799397, 0.006612473344882377653 ) ) ;
#6310=CARTESIAN_POINT ( 'NONE',  ( -4.177541715523163113, 56.60546344811582742, -4.746664548824306884 ) ) ;
#6311=CARTESIAN_POINT ( 'NONE',  ( -15.49691217297365142, 66.69002736867275871, 7.815521802502809479 ) ) ;
#6315=CARTESIAN_POINT ( 'NONE',  ( -33.76207074264209496, 50.00000000000002842, -7.785926851161516095E-15 ) ) ;
#6319=ORIENTED_EDGE ( 'NONE', *, *, #6109, .T. ) ;
#6324=EDGE_CURVE ( 'NONE', #3266, #9403, #2266, .T. ) ;
#6326=CARTESIAN_POINT ( 'NONE',  ( -45.57393268948897713, 54.97518271910073651, 0.008495404467763291445 ) ) ;
#6332=CARTESIAN_POINT ( 'NONE',  ( -61.00490302436042356, 55.00059028654953153, 21.02810969917934614 ) ) ;
#6334=CARTESIAN_POINT ( 'NONE',  ( -43.99614436914441029, 63.04465853171391387, -19.42287488623002290 ) ) ;
#6338=CARTESIAN_POINT ( 'NONE',  ( -21.05849041552747281, 57.05917194494736577, 20.98221040122819403 ) ) ;
#6339=CIRCLE ( 'NONE', #9379, 9.999999999999987566 ) ;
#6340=EDGE_LOOP ( 'NONE', ( #9997, #1248, #4796, #3548 ) ) ;
#6343=CARTESIAN_POINT ( 'NONE',  ( -62.54147003350998801, 53.97158195009890136, 6.934912854774474944 ) ) ;
#6345=CARTESIAN_POINT ( 'NONE',  ( 5.070642430964857894, 34.06762781005689078, -2.059172530961658865 ) ) ;
#6348=CARTESIAN_POINT ( 'NONE',  ( -22.50647595179652072, 59.12487335784310005, 20.69694904210189179 ) ) ;
#6354=CARTESIAN_POINT ( 'NONE',  ( -43.04772718432226952, 54.99964267904652360, 0.005532449227661951838 ) ) ;
#6355=CARTESIAN_POINT ( 'NONE',  ( -35.67858024924570515, 51.94572111605872777, -3.972273510035316146 ) ) ;
#6357=CIRCLE ( 'NONE', #2714, 4.999999999999984013 ) ;
#6360=CARTESIAN_POINT ( 'NONE',  ( -55.53658087589213466, 59.34025876743092454, 2.504133036876110996 ) ) ;
#6364=CARTESIAN_POINT ( 'NONE',  ( -11.57142270279487306, 60.00000000000001421, -4.065933922700817035E-15 ) ) ;
#6365=CARTESIAN_POINT ( 'NONE',  ( 22.23809523809524435, 59.99999999999998579, 0.000000000000000000 ) ) ;
#6373=CARTESIAN_POINT ( 'NONE',  ( 4.036346099538457466, 42.32158391892036775, -5.996328608354988710 ) ) ;
#6381=CARTESIAN_POINT ( 'NONE',  ( -36.24052534987266938, 55.00849635663053050, 0.02481536697055203647 ) ) ;
#6387=ORIENTED_EDGE ( 'NONE', *, *, #10002, .T. ) ;
#6388=CARTESIAN_POINT ( 'NONE',  ( 3.737309610555803463, 34.06887424008940712, -2.059134394038261817 ) ) ;
#6393=CARTESIAN_POINT ( 'NONE',  ( -29.54809237377008202, 34.60091625530366599, 5.109976345715927515 ) ) ;
#6398=CARTESIAN_POINT ( 'NONE',  ( -0.7638017253321776057, 55.00780231169513002, 0.009546663813864672207 ) ) ;
#6400=CARTESIAN_POINT ( 'NONE',  ( -16.49360055079280940, 72.53723377933144434, 11.72566733603474098 ) ) ;
#6401=CARTESIAN_POINT ( 'NONE',  ( -34.17314261869798742, 34.29999169977881479, -4.109493429249395646 ) ) ;
#6407=CARTESIAN_POINT ( 'NONE',  ( -43.33118549350501780, 55.00018389033358091, -0.001986509158416555499 ) ) ;
#6408=CARTESIAN_POINT ( 'NONE',  ( -41.12561409036811000, 56.30289684387001614, -4.871785110082141657 ) ) ;
#6414=CARTESIAN_POINT ( 'NONE',  ( -29.48439297115004010, 51.23129068170470646, 3.302108576988587174 ) ) ;
#6424=CARTESIAN_POINT ( 'NONE',  ( 12.12709278872420526, 46.41256629213580709, 11.17685062095174331 ) ) ;
#6428=CARTESIAN_POINT ( 'NONE',  ( 23.00000000000000000, 76.00000000000000000, 0.000000000000000000 ) ) ;
#6433=CARTESIAN_POINT ( 'NONE',  ( -51.57640054972269184, 55.00858919803477676, 0.004561873522476029598 ) ) ;
#6437=CARTESIAN_POINT ( 'NONE',  ( -11.57142270279487306, 60.00000000000001421, -4.065933922700817035E-15 ) ) ;
#6443=CARTESIAN_POINT ( 'NONE',  ( -7.030643242133587378, 62.08114452727563304, -19.79025909736091648 ) ) ;
#6448=CARTESIAN_POINT ( 'NONE',  ( -5.030643890195627854, 62.08057558410310861, -19.78873666113293694 ) ) ;
#6450=CARTESIAN_POINT ( 'NONE',  ( -67.52720549794999272, 34.02364409886038743, 2.748840581154547102 ) ) ;
#6454=CARTESIAN_POINT ( 'NONE',  ( 1.697306494461763959, 35.98764835359665426, -8.991780390316415961 ) ) ;
#6457=CARTESIAN_POINT ( 'NONE',  ( -44.50647629921198245, 66.71846839581321831, -17.55227556201471018 ) ) ;
#6460=CARTESIAN_POINT ( 'NONE',  ( -18.69730990872651333, 70.57397863033268948, 14.11552877426516339 ) ) ;
#6467=CARTESIAN_POINT ( 'NONE',  ( -59.09748447831353246, 54.99655739826935275, -0.01220661389743049260 ) ) ;
#6468=CARTESIAN_POINT ( 'NONE',  ( -37.04640917235918351, 52.93602743192931115, -4.557080977652598897 ) ) ;
#6486=CARTESIAN_POINT ( 'NONE',  ( -9.071371961462144640, 67.39181373483076243, -6.619190081737647446 ) ) ;
#6495=CARTESIAN_POINT ( 'NONE',  ( -33.90726341901891772, 55.01734440879120314, 0.01967313780937999038 ) ) ;
#6497=DIRECTION ( 'NONE',  ( 0.000000000000000000, 1.000000000000000000, 0.000000000000000000 ) ) ;
#6501=CARTESIAN_POINT ( 'NONE',  ( 10.20138320063666981, 50.66135930820338018, 2.506893722508881428 ) ) ;
#6505=CARTESIAN_POINT ( 'NONE',  ( 8.189038476963473201, 38.19597440261895827, 12.92108669627241646 ) ) ;
#6510=CARTESIAN_POINT ( 'NONE',  ( 47.00000000000000000, 55.00000000000000000, 0.000000000000000000 ) ) ;
#6511=CARTESIAN_POINT ( 'NONE',  ( -42.07074724807011989, 61.10209548959944215, -20.11061483308460751 ) ) ;
#6513=CARTESIAN_POINT ( 'NONE',  ( -48.14429339001110009, 75.47411806927735256, -5.508782930744743567 ) ) ;
#6517=CARTESIAN_POINT ( 'NONE',  ( -6.160267096003628318, 59.12214581854949103, -20.69010011304746044 ) ) ;
#6520=CARTESIAN_POINT ( 'NONE',  ( -55.30273887647248188, 69.12493077113425954, 15.58380738211564598 ) ) ;
#6521=CARTESIAN_POINT ( 'NONE',  ( -54.88146047731135013, 73.03677976846768161, 10.81065700633557825 ) ) ;
#6524=CARTESIAN_POINT ( 'NONE',  ( 36.99999999999999289, 55.00000000000000000, 0.000000000000000000 ) ) ;
#6528=CARTESIAN_POINT ( 'NONE',  ( -18.23626112837376567, 55.01086945185167565, 0.005850176292158671722 ) ) ;
#6529=CARTESIAN_POINT ( 'NONE',  ( -42.28847398866372487, 57.21383472543325155, -4.495207825519515588 ) ) ;
#6534=CARTESIAN_POINT ( 'NONE',  ( -0.4175868455413908609, 49.57342814860067648, -4.454705972034904704 ) ) ;
#6536=CARTESIAN_POINT ( 'NONE',  ( 4.595919313165082620, 34.88938507153989832, -6.102095433906166377 ) ) ;
#6540=CARTESIAN_POINT ( 'NONE',  ( -28.32521755090752791, 51.94774187383560360, 3.973893490808335205 ) ) ;
#6546=AXIS2_PLACEMENT_3D ( 'NONE', #871, #2626, #10988 ) ;
#6550=CARTESIAN_POINT ( 'NONE',  ( -53.41065706016718195, 65.82748300578383294, 8.886592616255020616 ) ) ;
#6557=AXIS2_PLACEMENT_3D ( 'NONE', #6510, #10137, #6574 ) ;
#6563=CARTESIAN_POINT ( 'NONE',  ( 2.915746493136800677, 49.57776560221653028, -4.450368587613543703 ) ) ;
#6568=CARTESIAN_POINT ( 'NONE',  ( 36.99999999999999289, 55.00000000000000000, 0.000000000000000000 ) ) ;
#6572=CARTESIAN_POINT ( 'NONE',  ( -18.69730990872651333, 70.57397863033268948, 14.11552877426516339 ) ) ;
#6574=DIRECTION ( 'NONE',  ( 0.000000000000000000, 1.000000000000000000, 0.000000000000000000 ) ) ;
#6575=CARTESIAN_POINT ( 'NONE',  ( -7.070747353360942178, 68.33360022464046324, -16.24461469319379603 ) ) ;
#6576=CARTESIAN_POINT ( 'NONE',  ( 47.00000000000000000, 55.00000000000000000, 0.000000000000000000 ) ) ;
#6579=CARTESIAN_POINT ( 'NONE',  ( -3.820070243736458426, 53.39331019270914425, -4.746214706174638920 ) ) ;
#6580=CARTESIAN_POINT ( 'NONE',  ( -7.030643242133587378, 62.08114452727563304, -19.79025909736091648 ) ) ;
#6582=CARTESIAN_POINT ( 'NONE',  ( -54.99627942256360313, 69.86586178386589552, 14.86494236827769200 ) ) ;
#6583=CARTESIAN_POINT ( 'NONE',  ( -63.32723919479404628, 46.95276866351182576, 19.42062151208882170 ) ) ;
#6585=CARTESIAN_POINT ( 'NONE',  ( 47.00000000000000000, 55.00000000000000000, 0.000000000000000000 ) ) ;
#6588=DIRECTION ( 'NONE',  ( 0.000000000000000000, 1.000000000000000000, 0.000000000000000000 ) ) ;
#6591=CARTESIAN_POINT ( 'NONE',  ( -56.75693999477515206, 54.99569681699411205, -0.004837550478154266538 ) ) ;
#6592=CARTESIAN_POINT ( 'NONE',  ( -60.95549686576197956, 52.78924107303826219, 4.487718700620877854 ) ) ;
#6593=EDGE_CURVE ( 'NONE', #10886, #11411, #6339, .T. ) ;
#6596=CARTESIAN_POINT ( 'NONE',  ( -67.53217105066197234, 42.78699024297431919, 7.034873537760521600 ) ) ;
#6598=CARTESIAN_POINT ( 'NONE',  ( 16.47760469315713294, 57.74566955740679930, 20.97627666568605420 ) ) ;
#6610=CARTESIAN_POINT ( 'NONE',  ( -40.87813363220659113, 57.05701126625427122, -13.86937383821729064 ) ) ;
#6619=CARTESIAN_POINT ( 'NONE',  ( 12.44324801771031908, 50.71611971558893828, 5.579753105726120488 ) ) ;
#6628=CARTESIAN_POINT ( 'NONE',  ( 22.18771278451687579, 76.01886845420673922, 2.750080521686579793 ) ) ;
#6632=CARTESIAN_POINT ( 'NONE',  ( -53.45210586504737904, 71.88419113761085555, 12.52116934359859002 ) ) ;
#6636=LINE ( 'NONE', #141, #9166 ) ;
#6639=CARTESIAN_POINT ( 'NONE',  ( -31.66281119664097332, 33.97723560729814096, 0.0005193846780039007571 ) ) ;
#6640=CARTESIAN_POINT ( 'NONE',  ( -60.69833702282029009, 56.03208645306531110, 20.99415308669729541 ) ) ;
#6644=CARTESIAN_POINT ( 'NONE',  ( -15.87853224631106919, 59.96722547271372861, 0.6578075836705260526 ) ) ;
#6646=ORIENTED_EDGE ( 'NONE', *, *, #149, .F. ) ;
#6649=CARTESIAN_POINT ( 'NONE',  ( 47.00000000000000000, 55.00000000000000000, 0.000000000000000000 ) ) ;
#6653=CARTESIAN_POINT ( 'NONE',  ( 6.776654365471205921, 48.89940868992559331, 3.518858988106267738 ) ) ;
#6655=CARTESIAN_POINT ( 'NONE',  ( 12.52240408941406535, 44.41801188983610871, 18.37272825892985040 ) ) ;
#6662=B_SPLINE_CURVE_WITH_KNOTS ( 'NONE', 3,
 ( #6106, #1712, #4637, #746, #11023, #4361, #8794, #2834, #6501, #10749, #10130, #5142, #8077, #7899, #3393, #4421, #9856, #11712, #3460, #5203, #6284, #6168, #7004, #573, #7067, #10626, #9739, #10691, #2615, #2503, #9799, #1593, #3512, #5261, #7181, #1649 ),
 .UNSPECIFIED., .F., .F.,
 ( 4, 2, 2, 2, 2, 2, 2, 2, 2, 2, 2, 2, 2, 2, 2, 2, 2, 4 ),
 ( 0.09712894785450570945, 0.09788736314146703754, 0.09864577842842835176, 0.1001626090023510079, 0.1016794395762736641, 0.1031962701501963064, 0.1047131007241189626, 0.1062299312980416049, 0.1077467618719642611, 0.1092635924458869034, 0.1107804230198095596, 0.1122972535937322158, 0.1138140841676548581, 0.1153309147415775143, 0.1168477453155001566, 0.1183645758894228128, 0.1198814064633454690, 0.1213982370372681113 ),
 .UNSPECIFIED. ) ;
#6665=AXIS2_PLACEMENT_3D ( 'NONE', #7695, #2959, #3136 ) ;
#6670=CARTESIAN_POINT ( 'NONE',  ( -40.58948485229369396, 56.37310121344063418, -13.95855491746121579 ) ) ;
#6680=CARTESIAN_POINT ( 'NONE',  ( -24.10991423831773517, 51.46493228316985835, 6.139939154236729202 ) ) ;
#6685=LINE ( 'NONE', #10316, #9509 ) ;
#6688=CARTESIAN_POINT ( 'NONE',  ( -32.99614454614441428, 33.97685596767119165, 0.0005149883856687357403 ) ) ;
#6700=CARTESIAN_POINT ( 'NONE',  ( 6.058385820703728442, 34.79737119409461599, 6.139092558150637480 ) ) ;
#6702=CARTESIAN_POINT ( 'NONE',  ( 22.85428395102741206, 76.02051159816545578, 2.750403924439354775 ) ) ;
#6703=AXIS2_PLACEMENT_3D ( 'NONE', #6524, #1953, #11771 ) ;
#6704=CARTESIAN_POINT ( 'NONE',  ( 16.46050413285405511, 62.04246480880237158, 12.21692500290179417 ) ) ;
#6706=DIRECTION ( 'NONE',  ( -1.000000000000000000, -6.033820786006286457E-17, -0.000000000000000000 ) ) ;
#6716=CARTESIAN_POINT ( 'NONE',  ( 19.22346612386121123, 61.13239903974351108, 3.531884177702926841 ) ) ;
#6718=CARTESIAN_POINT ( 'NONE',  ( -7.662811188708723797, 69.86483622371564195, -14.86557385339502169 ) ) ;
#6730=CARTESIAN_POINT ( 'NONE',  ( -51.66851517836372665, 67.95242035046020135, 5.365460588887749793 ) ) ;
#6733=DIRECTION ( 'NONE',  ( -6.033820786006286457E-17, 1.000000000000000000, 0.000000000000000000 ) ) ;
#6736=AXIS2_PLACEMENT_3D ( 'NONE', #5716, #9353, #4812 ) ;
#6740=CARTESIAN_POINT ( 'NONE',  ( -37.65876738585033934, 51.02620280256623886, -3.052412481529861665 ) ) ;
#6742=CARTESIAN_POINT ( 'NONE',  ( 3.500170968731791898, 49.14645465064588592, -3.907445888089149832 ) ) ;
#6747=AXIS2_PLACEMENT_3D ( 'NONE', #8890, #1577, #10608 ) ;
#6749=FACE_OUTER_BOUND ( 'NONE', #181, .T. ) ;
#6752=CARTESIAN_POINT ( 'NONE',  ( -50.14429338685609849, 75.46958046783008456, -5.506903914760000518 ) ) ;
#6755=CARTESIAN_POINT ( 'NONE',  ( -52.00383529082647271, 74.42722782460430153, 8.047526119559261559 ) ) ;
#6762=CARTESIAN_POINT ( 'NONE',  ( -17.27494751259140315, 73.62640980466187557, 9.944421848179040069 ) ) ;
#6764=CARTESIAN_POINT ( 'NONE',  ( -2.810961525112865012, 49.49246827230374635, -20.47109371692935298 ) ) ;
#6765=CARTESIAN_POINT ( 'NONE',  ( -59.82750509709391196, 59.10995506582904824, 20.69284243654335498 ) ) ;
#6773=CARTESIAN_POINT ( 'NONE',  ( -71.32904977408374236, 54.99618961743304624, -0.002957579938396712443 ) ) ;
#6775=CARTESIAN_POINT ( 'NONE',  ( 16.89002048584296745, 59.31391198272093845, 5.609897141675635801 ) ) ;
#6778=CARTESIAN_POINT ( 'NONE',  ( -22.47759590436300314, 52.25445647903773505, 21.02373912143526979 ) ) ;
#6784=ORIENTED_EDGE ( 'NONE', *, *, #6156, .T. ) ;
#6786=CARTESIAN_POINT ( 'NONE',  ( 47.00000000000000000, 50.00000000000000000, 0.000000000000000000 ) ) ;
#6787=CARTESIAN_POINT ( 'NONE',  ( -64.86550693891295793, 42.79548891016047918, 7.031200541850135544 ) ) ;
#6796=CARTESIAN_POINT ( 'NONE',  ( -52.03951664420899448, 59.99999999999998579, -0.3298728053696415308 ) ) ;
#6799=CARTESIAN_POINT ( 'NONE',  ( -18.66680221850326760, 57.68121094790071623, 6.472159763528865462 ) ) ;
#6805=CARTESIAN_POINT ( 'NONE',  ( -21.63602683877659771, 62.08561388645346568, 19.80191166437241179 ) ) ;
#6809=CARTESIAN_POINT ( 'NONE',  ( -48.14429339001110009, 75.47411806927735256, -5.508782930744743567 ) ) ;
#6817=CARTESIAN_POINT ( 'NONE',  ( -26.81096152405270061, 44.41979049410412017, 18.36814973051028588 ) ) ;
#6819=CARTESIAN_POINT ( 'NONE',  ( -8.996144538211344965, 69.86510777810948980, -14.86583919048846170 ) ) ;
#6820=CARTESIAN_POINT ( 'NONE',  ( -42.36967124068387136, 54.31236102449236824, -13.99392387036892238 ) ) ;
#6821=DIRECTION ( 'NONE',  ( 1.000000000000000000, 6.033820786006286457E-17, 0.000000000000000000 ) ) ;
#6829=AXIS2_PLACEMENT_3D ( 'NONE', #6576, #10206, #5980 ) ;
#6833=CARTESIAN_POINT ( 'NONE',  ( -39.10991423111748588, 50.68603547566416978, -5.609840947021430324 ) ) ;
#6835=CARTESIAN_POINT ( 'NONE',  ( -13.85565285731654761, 75.43037139504293975, 5.490367781071763709 ) ) ;
#6837=CARTESIAN_POINT ( 'NONE',  ( 0.000000000000000000, 0.000000000000000000, 0.000000000000000000 ) ) ;
#6843=EDGE_LOOP ( 'NONE', ( #2634, #2556 ) ) ;
#6846=CARTESIAN_POINT ( 'NONE',  ( 52.99999999999999289, 58.53553390593273065, 3.535533905932731091 ) ) ;
#6848=CARTESIAN_POINT ( 'NONE',  ( 14.14423903981857755, 49.50929293985068114, 20.43023407247793699 ) ) ;
#6849=AXIS2_PLACEMENT_3D ( 'NONE', #4090, #7040, #9656 ) ;
#6859=CARTESIAN_POINT ( 'NONE',  ( -42.70536343102052257, 54.67063349880791634, -5.000011853200844847 ) ) ;
#6861=CARTESIAN_POINT ( 'NONE',  ( -51.04203483874748315, 61.59087299007505578, 2.357793790660874134 ) ) ;
#6871=CARTESIAN_POINT ( 'NONE',  ( -64.47562408583945626, 38.19583575827792288, 12.92744520505189953 ) ) ;
#6875=CARTESIAN_POINT ( 'NONE',  ( -39.18898618735786243, 44.43394377878069434, -18.33326528472845141 ) ) ;
#6877=CARTESIAN_POINT ( 'NONE',  ( -18.33720990162648690, 69.86853815246008992, 14.86915066445586042 ) ) ;
#6878=CARTESIAN_POINT ( 'NONE',  ( -43.54480028671723346, 57.05700836894583716, -13.86810795104769412 ) ) ;
#6888=CARTESIAN_POINT ( 'NONE',  ( -22.29127922628105551, 57.36276450979780606, 6.604096906534940636 ) ) ;
#6891=CARTESIAN_POINT ( 'NONE',  ( -52.00383529082647271, 74.42722782460430153, 8.047526119559261559 ) ) ;
#6893=FACE_OUTER_BOUND ( 'NONE', #5864, .T. ) ;
#6903=CARTESIAN_POINT ( 'NONE',  ( -24.81096152833125856, 44.41791055217656492, 18.37268719335390443 ) ) ;
#6912=DIRECTION ( 'NONE',  ( -1.000000000000000000, 0.000000000000000000, 0.000000000000000000 ) ) ;
#6916=CARTESIAN_POINT ( 'NONE',  ( -63.77645048510821368, 49.38553753369352961, 4.319276899024868221 ) ) ;
#6930=CARTESIAN_POINT ( 'NONE',  ( 8.496464703907626870, 55.00583224785918901, 0.0002657300979511648576 ) ) ;
#6936=CARTESIAN_POINT ( 'NONE',  ( -15.85565286160008469, 75.43490621471428881, 5.492246195135631837 ) ) ;
#6938=CARTESIAN_POINT ( 'NONE',  ( 2.363972944155686928, 35.98715435331354939, -8.992005631236420271 ) ) ;
#6939=CARTESIAN_POINT ( 'NONE',  ( -10.29698636593376371, 65.39011648954584643, -9.417152705430359205 ) ) ;
#6943=CARTESIAN_POINT ( 'NONE',  ( -20.53797830674339764, 58.05056462116689175, 3.975025670360801566 ) ) ;
#6949=CARTESIAN_POINT ( 'NONE',  ( -42.99986031074618609, 55.00026768892313100, -7.010501145347482144 ) ) ;
#6951=CARTESIAN_POINT ( 'NONE',  ( -32.17314280228392676, 34.29902663375150240, -4.109485608336678197 ) ) ;
#6953=CARTESIAN_POINT ( 'NONE',  ( 5.506399570602333426, 34.30736306936326230, 4.109392375493936100 ) ) ;
#6963=CARTESIAN_POINT ( 'NONE',  ( 6.329456780446692576, 33.97189653527247089, -0.0004287163746460355418 ) ) ;
#6971=CARTESIAN_POINT ( 'NONE',  ( -68.74447550303376886, 50.00000002723004400, -0.0005274282990175871997 ) ) ;
#6975=CARTESIAN_POINT ( 'NONE',  ( -31.49982903124580602, 48.09671445454723937, -1.369954454670364807 ) ) ;
#6977=CARTESIAN_POINT ( 'NONE',  ( 62.44550000000000267, 55.00000000000000000, 0.000000000000000000 ) ) ;
#6987=FACE_OUTER_BOUND ( 'NONE', #4160, .T. ) ;
#6992=CARTESIAN_POINT ( 'NONE',  ( -53.69727390230763575, 74.79022971164903311, 7.081167078663678893 ) ) ;
#6993=EDGE_LOOP ( 'NONE', ( #4007, #9657, #5824, #10969 ) ) ;
#6994=CARTESIAN_POINT ( 'NONE',  ( -26.85565286017724418, 42.10688304539454663, 16.77644304551772336 ) ) ;
#6995=CARTESIAN_POINT ( 'NONE',  ( 0.4968476615399680107, 43.29813335323204626, -7.812534750456064714 ) ) ;
#7004=CARTESIAN_POINT ( 'NONE',  ( 18.37142430252887237, 56.60669449543473775, 4.746147407754762071 ) ) ;
#7005=CARTESIAN_POINT ( 'NONE',  ( -55.54150741847631423, 61.01381665909754304, 3.604391452501248150 ) ) ;
#7007=CARTESIAN_POINT ( 'NONE',  ( -50.27495406422890767, 76.01781437481966464, 2.059423474151367728 ) ) ;
#7008=CARTESIAN_POINT ( 'NONE',  ( 17.52230480588388417, 67.92092721363508190, 16.80419350660125843 ) ) ;
#7009=CARTESIAN_POINT ( 'NONE',  ( 37.00000000000000000, 50.00000000000000000, 0.000000000000000000 ) ) ;
#7011=APPLICATION_CONTEXT ( 'automotive_design' ) ;
#7013=VERTEX_POINT ( 'NONE', #8166 ) ;
#7017=VECTOR ( 'NONE', #1298, 1000.000000000000114 ) ;
#7018=CARTESIAN_POINT ( 'NONE',  ( -7.662811188708723797, 69.86483622371564195, -14.86557385339502169 ) ) ;
#7022=CARTESIAN_POINT ( 'NONE',  ( -71.09399662003431786, 50.00000004634800632, -0.0006807936302138478625 ) ) ;
#7025=CARTESIAN_POINT ( 'NONE',  ( -44.96936008568403764, 63.99178041037959019, -19.01235157881157178 ) ) ;
#7034=EDGE_LOOP ( 'NONE', ( #4396, #9555, #6387, #10015, #8015, #4384 ) ) ;
#7036=CARTESIAN_POINT ( 'NONE',  ( -47.44324763638165621, 61.84126198528888096, -1.841921628722773097 ) ) ;
#7040=DIRECTION ( 'NONE',  ( 1.000000000000000000, 6.033820786006286457E-17, 0.000000000000000000 ) ) ;
#7049=CARTESIAN_POINT ( 'NONE',  ( 4.714426611521913557, 54.99241905126812924, -0.004073598914535226517 ) ) ;
#7054=CARTESIAN_POINT ( 'NONE',  ( -27.51876704757110303, 50.51322248963012385, 2.212644460676499669 ) ) ;
#7058=CARTESIAN_POINT ( 'NONE',  ( -38.52231951926622600, 44.43456989975021543, -18.33175367071157780 ) ) ;
#7059=CARTESIAN_POINT ( 'NONE',  ( -33.33147340253317736, 40.98517796169446825, 0.0004158008307579650481 ) ) ;
#7061=ORIENTED_EDGE ( 'NONE', *, *, #7133, .F. ) ;
#7063=CARTESIAN_POINT ( 'NONE',  ( 63.00000000000000000, 55.00000000000000000, 0.000000000000000000 ) ) ;
#7067=CARTESIAN_POINT ( 'NONE',  ( 19.52954336140098235, 57.50311058138565556, 4.340816333004676508 ) ) ;
#7068=CARTESIAN_POINT ( 'NONE',  ( -33.66680225892029910, 47.99349995571937910, 0.0003166132758461101537 ) ) ;
#7070=CARTESIAN_POINT ( 'NONE',  ( -6.003876560668130580, 63.04743182124521184, -19.42709301306817693 ) ) ;
#7074=CARTESIAN_POINT ( 'NONE',  ( 63.00000000000000000, 55.00000000000000000, -2.445500000000003116 ) ) ;
#7080=CARTESIAN_POINT ( 'NONE',  ( 3.697305843545918513, 35.98616635274733255, -8.992456113074794644 ) ) ;
#7086=CARTESIAN_POINT ( 'NONE',  ( 36.99999999999999289, 55.00000000000000000, 0.000000000000000000 ) ) ;
#7087=CARTESIAN_POINT ( 'NONE',  ( -54.59603348275399526, 73.54984634329692028, 9.912388241271610667 ) ) ;
#7095=ORIENTED_EDGE ( 'NONE', *, *, #8813, .T. ) ;
#7096=CARTESIAN_POINT ( 'NONE',  ( -28.87484158014380853, 48.19745421759348858, 1.704321637862361349 ) ) ;
#7108=CARTESIAN_POINT ( 'NONE',  ( 5.871464932984317819, 55.00507431483917031, 0.002345699056559674180 ) ) ;
#7111=EDGE_LOOP ( 'NONE', ( #274, #1567 ) ) ;
#7116=CARTESIAN_POINT ( 'NONE',  ( -42.26269064503769357, 57.05915346985771208, -20.93174897424885472 ) ) ;
#7117=CARTESIAN_POINT ( 'NONE',  ( -46.16981911518406179, 62.81253473440293078, -11.70186679652239725 ) ) ;
#7119=AXIS2_PLACEMENT_3D ( 'NONE', #7211, #2464, #6132 ) ;
#7123=DIRECTION ( 'NONE',  ( -1.000000000000000000, -0.000000000000000000, -0.000000000000000000 ) ) ;
#7128=CARTESIAN_POINT ( 'NONE',  ( 0.7144279133528070869, 54.99538305296515261, -0.002722153396144796379 ) ) ;
#7130=CARTESIAN_POINT ( 'NONE',  ( -68.34104732181945963, 33.99448141944315438, 0.006743540747239065887 ) ) ;
#7131=CARTESIAN_POINT ( 'NONE',  ( -17.82693376281896391, 72.53768310958322729, 11.72612467905221934 ) ) ;
#7133=EDGE_CURVE ( 'NONE', #10196, #2759, #835, .T. ) ;
#7138=FACE_OUTER_BOUND ( 'NONE', #10773, .T. ) ;
#7140=CARTESIAN_POINT ( 'NONE',  ( -31.30269415623623885, 33.99224428815358579, -1.031667027462585207 ) ) ;
#7147=CARTESIAN_POINT ( 'NONE',  ( 16.79625880786201719, 58.05269072103210704, 3.973457567300640036 ) ) ;
#7149=CARTESIAN_POINT ( 'NONE',  ( 36.99999999999999289, 55.00000000000000000, 0.000000000000000000 ) ) ;
#7152=VERTEX_POINT ( 'NONE', #7572 ) ;
#7154=CARTESIAN_POINT ( 'NONE',  ( 15.20622923973939677, 53.16901270175023342, 14.02455805003628520 ) ) ;
#7156=CARTESIAN_POINT ( 'NONE',  ( 53.00000000000000000, 51.46446609406726935, 3.535533905932731091 ) ) ;
#7164=CARTESIAN_POINT ( 'NONE',  ( -0.4260572601936686854, 54.99150886132364491, -0.02483499414063310151 ) ) ;
#7167=ORIENTED_EDGE ( 'NONE', *, *, #5230, .T. ) ;
#7170=CARTESIAN_POINT ( 'NONE',  ( -67.17448730496187181, 36.66801277209461318, 10.55271442276269944 ) ) ;
#7172=CARTESIAN_POINT ( 'NONE',  ( -41.36397681821770078, 53.96873918909963663, -20.99311060721154121 ) ) ;
#7181=CARTESIAN_POINT ( 'NONE',  ( 25.37133272033247877, 59.99999999999997158, 0.3324664797073844102 ) ) ;
#7182=CARTESIAN_POINT ( 'NONE',  ( 4.496465067834011009, 55.00390890337079242, 0.0002487324669923884337 ) ) ;
#7184=CARTESIAN_POINT ( 'NONE',  ( 8.811013807768157236, 36.66975794146507184, 10.56480398736207960 ) ) ;
#7185=CARTESIAN_POINT ( 'NONE',  ( -38.47762819156672265, 42.07891330237754346, -16.80402559754432801 ) ) ;
#7189=EDGE_LOOP ( 'NONE', ( #7238, #9695, #11164, #290 ) ) ;
#7193=EDGE_CURVE ( 'NONE', #1626, #9767, #1329, .T. ) ;
#7194=AXIS2_PLACEMENT_3D ( 'NONE', #6585, #1292, #2976 ) ;
#7196=CARTESIAN_POINT ( 'NONE',  ( -53.73751484135783585, 71.24472392590685388, 13.33357819947211453 ) ) ;
#7204=ADVANCED_FACE ( 'NONE', ( #8522 ), #10545, .F. ) ;
#7211=CARTESIAN_POINT ( 'NONE',  ( 52.99999999999999289, 55.00000000000000000, 0.000000000000000000 ) ) ;
#7214=CARTESIAN_POINT ( 'NONE',  ( 17.53948780091567983, 58.67519633682641000, 13.65775887405797029 ) ) ;
#7224=LINE ( 'NONE', #3612, #5786 ) ;
#7225=CARTESIAN_POINT ( 'NONE',  ( -41.95224010427075001, 55.00407356838249484, -0.007580890217307994366 ) ) ;
#7230=CARTESIAN_POINT ( 'NONE',  ( -13.12643311661332746, 59.84143854988970190, 1.290711584744844043 ) ) ;
#7232=CARTESIAN_POINT ( 'NONE',  ( -65.06671514604981610, 41.61929618219224380, 16.30332023460171698 ) ) ;
#7234=CARTESIAN_POINT ( 'NONE',  ( -19.78535886778656661, 65.80747357543212672, 18.02991983063459003 ) ) ;
#7238=ORIENTED_EDGE ( 'NONE', *, *, #5200, .T. ) ;
#7240=CARTESIAN_POINT ( 'NONE',  ( -25.52231952398968673, 42.10919693116569817, 16.77412918608628090 ) ) ;
#7243=CARTESIAN_POINT ( 'NONE',  ( 20.42601516676554851, 54.98551770566741936, -0.007780136594349751702 ) ) ;
#7246=CARTESIAN_POINT ( 'NONE',  ( -59.00490307935969270, 55.00061426705308065, 21.02882928537637497 ) ) ;
#7247=CARTESIAN_POINT ( 'NONE',  ( -24.47759590008010377, 52.25445690686086664, 21.01882782503509262 ) ) ;
#7248=( NAMED_UNIT ( * ) PLANE_ANGLE_UNIT ( ) SI_UNIT ( $, .RADIAN. ) );
#7252=CARTESIAN_POINT ( 'NONE',  ( -93.29762528721818171, 110.0087426977633669, -0.02929211074601270615 ) ) ;
#7253=DIRECTION ( 'NONE',  ( 1.000000000000000000, 0.000000000000000000, -0.000000000000000000 ) ) ;
#7254=CARTESIAN_POINT ( 'NONE',  ( -54.34438039152910704, 58.05280871788295372, 3.973341673354612524 ) ) ;
#7257=CARTESIAN_POINT ( 'NONE',  ( -55.14769694417690715, 59.49448256121726786, 2.215039651009127031 ) ) ;
#7268=CARTESIAN_POINT ( 'NONE',  ( -12.79377121657755190, 69.02455796469044458, 1.830988287285042926 ) ) ;
#7274=AXIS2_PLACEMENT_3D ( 'NONE', #7791, #4191, #4813 ) ;
#7275=ORIENTED_EDGE ( 'NONE', *, *, #2800, .T. ) ;
#7280=CARTESIAN_POINT ( 'NONE',  ( -63.42686368473390957, 54.98038842139913385, 0.01519274601354845579 ) ) ;
#7284=CARTESIAN_POINT ( 'NONE',  ( -14.68353320191416067, 59.33897812137291794, 2.505989342657766628 ) ) ;
#7288=CARTESIAN_POINT ( 'NONE',  ( 12.85570563148687739, 52.25434904275299175, 21.01882863504484789 ) ) ;
#7293=CARTESIAN_POINT ( 'NONE',  ( 0.1442708919848544047, 44.43605983923426805, -18.32883121229183487 ) ) ;
#7295=ADVANCED_FACE ( 'NONE', ( #11737 ), #3486, .T. ) ;
#7299=CARTESIAN_POINT ( 'NONE',  ( -10.09032851302145950, 54.99509807286066376, 0.004314335854857118992 ) ) ;
#7301=CARTESIAN_POINT ( 'NONE',  ( -59.36500404872999326, 56.03206174438126652, 20.99316529255160191 ) ) ;
#7303=CARTESIAN_POINT ( 'NONE',  ( 3.451907635234679361, 34.19915017745972108, -3.085386652995293133 ) ) ;
#7308=ORIENTED_EDGE ( 'NONE', *, *, #8281, .F. ) ;
#7310=CARTESIAN_POINT ( 'NONE',  ( -51.90718173048562534, 54.98364889560268409, -0.001639402367017143113 ) ) ;
#7311=CARTESIAN_POINT ( 'NONE',  ( -38.01415270387070677, 53.70170271778372495, -4.839460789004083274 ) ) ;
#7319=CARTESIAN_POINT ( 'NONE',  ( 21.84682584988675202, 59.99999999999999289, 0.3320659484734538869 ) ) ;
#7324=FACE_BOUND ( 'NONE', #3196, .T. ) ;
#7326=LINE ( 'NONE', #10053, #10275 ) ;
#7327=CARTESIAN_POINT ( 'NONE',  ( 22.20627439270837655, 67.25635803115373790, 7.058475852763654856 ) ) ;
#7331=LINE ( 'NONE', #6428, #1289 ) ;
#7336=CARTESIAN_POINT ( 'NONE',  ( -57.71391471235212123, 54.99984036959516942, -0.007998007078910979867 ) ) ;
#7341=CARTESIAN_POINT ( 'NONE',  ( -24.79786866689667946, 51.95154789264624640, 3.976631450565629500 ) ) ;
#7345=CARTESIAN_POINT ( 'NONE',  ( 2.595920079249742329, 34.88763922991881827, -6.102757042485290384 ) ) ;
#7349=EDGE_CURVE ( 'NONE', #4551, #1195, #10345, .T. ) ;
#7351=CARTESIAN_POINT ( 'NONE',  ( -38.60828084422895046, 48.85949782923615459, -20.20603288453101243 ) ) ;
#7354=CARTESIAN_POINT ( 'NONE',  ( 13.42607030714540706, 55.00164660868858135, -0.01635937553770835245 ) ) ;
#7356=CARTESIAN_POINT ( 'NONE',  ( -25.47762819357030395, 44.41853719948864665, 18.37117470573356925 ) ) ;
#7357=CARTESIAN_POINT ( 'NONE',  ( -32.11869219899978845, 34.20636958863568822, 3.085052597841025701 ) ) ;
#7362=ORIENTED_EDGE ( 'NONE', *, *, #8927, .F. ) ;
#7364=CARTESIAN_POINT ( 'NONE',  ( -56.46182468818901157, 54.99756168373090048, -0.002722472456010964752 ) ) ;
#7365=CARTESIAN_POINT ( 'NONE',  ( -60.76133702166824690, 52.93822791804927164, 4.558078328184683947 ) ) ;
#7366=CYLINDRICAL_SURFACE ( 'NONE', #3856, 4.999999999999984013 ) ;
#7369=CARTESIAN_POINT ( 'NONE',  ( 21.14436220910852882, 71.77416011014268804, 12.89076390558360075 ) ) ;
#7379=CARTESIAN_POINT ( 'NONE',  ( 3.163514083425913892, 43.29694055639052408, -7.813017536009592590 ) ) ;
#7389=CARTESIAN_POINT ( 'NONE',  ( -53.61888101636234438, 55.00545574595133047, 0.006701513939034802261 ) ) ;
#7393=CARTESIAN_POINT ( 'NONE',  ( 47.00000000000000000, 55.00000000000000000, 0.000000000000000000 ) ) ;
#7400=CARTESIAN_POINT ( 'NONE',  ( -69.67438043473205767, 33.99524309754638551, 0.006656162479001280670 ) ) ;
#7405=CARTESIAN_POINT ( 'NONE',  ( -40.03064391692543467, 53.96877717286832876, -20.99202776130344361 ) ) ;
#7414=CARTESIAN_POINT ( 'NONE',  ( -19.40408043161419371, 64.90577468530469218, 18.53575269199317788 ) ) ;
#7416=CARTESIAN_POINT ( 'NONE',  ( -52.27495405780593529, 76.01412898031726684, 2.059423305703688811 ) ) ;
#7426=CARTESIAN_POINT ( 'NONE',  ( -34.00213111530580079, 55.00182194974264860, 0.0002174257210376325542 ) ) ;
#7427=CARTESIAN_POINT ( 'NONE',  ( -34.51742062993405824, 51.23169754889989491, -3.302621543381780711 ) ) ;
#7431=CARTESIAN_POINT ( 'NONE',  ( -9.458587434131468186, 59.17210302956776502, -5.626626392890127448 ) ) ;
#7444=DIRECTION ( 'NONE',  ( 1.000000000000000000, 6.033820786006286457E-17, 0.000000000000000000 ) ) ;
#7445=CARTESIAN_POINT ( 'NONE',  ( -43.50315269332450185, 62.81301754493210154, -11.70305962917251819 ) ) ;
#7456=CARTESIAN_POINT ( 'NONE',  ( -60.61922519846778101, 54.99654146924289222, 0.007592002550234120892 ) ) ;
#7463=ADVANCED_FACE ( 'NONE', ( #7324, #5580 ), #9223, .T. ) ;
#7466=ORIENTED_EDGE ( 'NONE', *, *, #9828, .T. ) ;
#7467=CARTESIAN_POINT ( 'NONE',  ( -63.84363901113670892, 43.28205526181564267, 17.55452879243513920 ) ) ;
#7473=CARTESIAN_POINT ( 'NONE',  ( -4.160267277967630406, 59.12176995062825569, -20.68921489609442332 ) ) ;
#7475=CARTESIAN_POINT ( 'NONE',  ( -32.72515708217407138, 34.82695427582095959, -6.127117481167428714 ) ) ;
#7477=CARTESIAN_POINT ( 'NONE',  ( 36.99999999999999289, 64.99999999999998579, 0.000000000000000000 ) ) ;
#7479=CARTESIAN_POINT ( 'NONE',  ( 7.477680471578420196, 36.66673471410030061, 10.56605622896702990 ) ) ;
#7481=CARTESIAN_POINT ( 'NONE',  ( -39.27494750982320681, 48.85996770079779594, -20.20489819083377014 ) ) ;
#7482=CARTESIAN_POINT ( 'NONE',  ( -47.81092963715463640, 71.80394787507084686, -12.92116392654651058 ) ) ;
#7487=ORIENTED_EDGE ( 'NONE', *, *, #9461, .T. ) ;
#7489=CARTESIAN_POINT ( 'NONE',  ( -42.17020159496552623, 54.99975127115207840, 0.003908898248491586742 ) ) ;
#7490=CARTESIAN_POINT ( 'NONE',  ( -47.34878363292850878, 59.83931338121328025, -1.298758957765639321 ) ) ;
#7494=CARTESIAN_POINT ( 'NONE',  ( 9.890116692599228543, 51.46809947807167873, 6.132390081685909600 ) ) ;
#7496=CARTESIAN_POINT ( 'NONE',  ( 5.451907626115248817, 34.19820075889870026, -3.085388827037094828 ) ) ;
#7508=CARTESIAN_POINT ( 'NONE',  ( -48.53950828781236737, 68.97547034813443645, -1.831174528873022345 ) ) ;
#7516=CARTESIAN_POINT ( 'NONE',  ( -35.70892724115440586, 50.25524874376613838, -1.610804148112624290 ) ) ;
#7518=CARTESIAN_POINT ( 'NONE',  ( -15.16689040116921916, 60.84304562314972742, 3.905604940474681985 ) ) ;
#7520=CYLINDRICAL_SURFACE ( 'NONE', #8924, 4.999999999999997335 ) ;
#7525=CARTESIAN_POINT ( 'NONE',  ( -3.477628190354089099, 49.49309465598528845, -20.46958112014059950 ) ) ;
#7528=CARTESIAN_POINT ( 'NONE',  ( -57.27472358375123207, 61.14040963541170015, 20.20590277145669234 ) ) ;
#7529=CARTESIAN_POINT ( 'NONE',  ( -57.27472358375123207, 61.14040963541170015, 20.20590277145669234 ) ) ;
#7532=FACE_OUTER_BOUND ( 'NONE', #2737, .T. ) ;
#7533=ADVANCED_FACE ( 'NONE', ( #10876 ), #10038, .T. ) ;
#7536=CARTESIAN_POINT ( 'NONE',  ( -57.94139028520521606, 61.13994508777751236, 20.20477452650387207 ) ) ;
#7537=CARTESIAN_POINT ( 'NONE',  ( -69.52691976458234535, 34.01892180236649921, 2.749684864678113794 ) ) ;
#7549=CARTESIAN_POINT ( 'NONE',  ( -66.79270227826378914, 43.79499200241600931, 8.618888393567598172 ) ) ;
#7550=ORIENTED_EDGE ( 'NONE', *, *, #4803, .T. ) ;
#7551=FACE_OUTER_BOUND ( 'NONE', #6993, .T. ) ;
#7563=CARTESIAN_POINT ( 'NONE',  ( -62.74205264515926928, 46.08327288479434003, 10.86410523659212934 ) ) ;
#7572=CARTESIAN_POINT ( 'NONE',  ( 46.99999999999999289, 58.53553390593273065, 3.535533905932731091 ) ) ;
#7574=CARTESIAN_POINT ( 'NONE',  ( -21.77654998131960795, 54.08371276951305617, 7.025374987337092314 ) ) ;
#7583=CARTESIAN_POINT ( 'NONE',  ( -36.14426256656389569, 36.63180902967581432, -10.58010824564746599 ) ) ;
#7590=CARTESIAN_POINT ( 'NONE',  ( -10.04436138461520933, 58.30566320991975005, -3.765552063897302126 ) ) ;
#7593=VERTEX_POINT ( 'NONE', #997 ) ;
#7594=CARTESIAN_POINT ( 'NONE',  ( 11.18907075893384828, 44.41926513478889404, 18.36970340340424457 ) ) ;
#7595=CARTESIAN_POINT ( 'NONE',  ( 5.737947948793154396, 41.52763994192435604, 4.093911426704439194 ) ) ;
#7596=CARTESIAN_POINT ( 'NONE',  ( 52.99999999999999289, 58.53553390593273065, 3.535533905932731091 ) ) ;
#7600=EDGE_CURVE ( 'NONE', #1442, #3266, #10159, .T. ) ;
#7602=CARTESIAN_POINT ( 'NONE',  ( 47.00000000000000000, 58.53553390593273065, -3.535533905932743526 ) ) ;
#7606=CARTESIAN_POINT ( 'NONE',  ( 1.916198795564182600, 48.29978761853648450, -2.032333837344214800 ) ) ;
#7609=CARTESIAN_POINT ( 'NONE',  ( 3.697305843545918513, 35.98616635274733255, -8.992456113074794644 ) ) ;
#7610=LINE ( 'NONE', #283, #1363 ) ;
#7611=CARTESIAN_POINT ( 'NONE',  ( 52.99999999999999289, 55.00000000000000000, 0.000000000000000000 ) ) ;
#7620=CARTESIAN_POINT ( 'NONE',  ( 19.52230480204648799, 67.92440004991483704, 16.80766691833610693 ) ) ;
#7624=VECTOR ( 'NONE', #2343, 1000.000000000000000 ) ;
#7628=CARTESIAN_POINT ( 'NONE',  ( -43.29000404689811177, 55.16495308597901470, -4.999994068545482229 ) ) ;
#7631=CARTESIAN_POINT ( 'NONE',  ( 24.88735338357604476, 62.02547980208617417, 0.9195476851153630005 ) ) ;
#7640=CARTESIAN_POINT ( 'NONE',  ( -33.30269350532120143, 33.99387206627966407, -1.031609878214063025 ) ) ;
#7643=CARTESIAN_POINT ( 'NONE',  ( -53.73751484135783585, 71.24472392590685388, 13.33357819947211453 ) ) ;
#7649=CARTESIAN_POINT ( 'NONE',  ( -7.320490228006724998, 56.29691533456504970, -4.839845655098152122 ) ) ;
#7650=CARTESIAN_POINT ( 'NONE',  ( 10.52240409369262153, 44.41989175727180594, 18.36819097564579195 ) ) ;
#7652=CARTESIAN_POINT ( 'NONE',  ( 6.725052486299625265, 34.79623650017382630, 6.139562429837428503 ) ) ;
#7653=CARTESIAN_POINT ( 'NONE',  ( -61.88037028687247698, 51.91449295574040690, 20.80032498971814192 ) ) ;
#7656=CIRCLE ( 'NONE', #7274, 4.999999999999990230 ) ;
#7665=CARTESIAN_POINT ( 'NONE',  ( -7.708699213456044141, 57.35874996863078934, -6.593436642072879827 ) ) ;
#7667=CARTESIAN_POINT ( 'NONE',  ( -40.33720992201957500, 55.00042869323097960, -21.02810349118288258 ) ) ;
#7671=CARTESIAN_POINT ( 'NONE',  ( 52.99999999999999289, 55.00000000000000000, -3.000000000000002665 ) ) ;
#7677=CARTESIAN_POINT ( 'NONE',  ( -45.46040646759425385, 66.21151220796895132, -8.622207064378679675 ) ) ;
#7678=EDGE_CURVE ( 'NONE', #8851, #1911, #5774, .T. ) ;
#7685=LINE ( 'NONE', #11375, #10322 ) ;
#7686=CARTESIAN_POINT ( 'NONE',  ( -41.54352521660307929, 53.70653700278867859, -4.840732458542600369 ) ) ;
#7689=CARTESIAN_POINT ( 'NONE',  ( 14.77655085292736281, 53.17745613723639053, 6.794376823515287711 ) ) ;
#7695=CARTESIAN_POINT ( 'NONE',  ( 34.00000000000000000, 55.00000000000000000, 0.000000000000000000 ) ) ;
#7698=CARTESIAN_POINT ( 'NONE',  ( -65.06671514604981610, 41.61929618219224380, 16.30332023460171698 ) ) ;
#7704=CARTESIAN_POINT ( 'NONE',  ( -57.82750524721426189, 59.10997802641301035, 20.69196764327204008 ) ) ;
#7709=B_SPLINE_CURVE_WITH_KNOTS ( 'NONE', 3,
 ( #6365, #7319, #8148, #5512, #3533, #9823, #882, #11672, #10830, #943, #7147, #10946, #3595, #8206, #11842, #1844, #10770, #2582, #4610, #8265, #40, #2524, #6248, #6190, #1612, #9875, #1671, #5339, #8991, #5573, #1007, #8506, #9219, #4667 ),
 .UNSPECIFIED., .F., .F.,
 ( 4, 2, 2, 2, 2, 2, 2, 2, 2, 2, 2, 2, 2, 2, 2, 2, 4 ),
 ( 0.000000000000000000, 0.001517779093106276078, 0.003035558186212552155, 0.004553337279318827799, 0.006071116372425104310, 0.007588895465531380821, 0.009106674558637655598, 0.01062445365174393211, 0.01214223274485020862, 0.01366001183795648513, 0.01517779093106276164, 0.01669557002416903815, 0.01821334911727531120, 0.01973112821038158771, 0.02124890730348786422, 0.02276668639659414073, 0.02428446548970041724 ),
 .UNSPECIFIED. ) ;
#7711=CARTESIAN_POINT ( 'NONE',  ( -20.73741325422386339, 64.90628579765783002, 18.53688757488948369 ) ) ;
#7714=CARTESIAN_POINT ( 'NONE',  ( -65.84115524907865336, 36.67226210568770028, 10.55087792480968112 ) ) ;
#7715=CARTESIAN_POINT ( 'NONE',  ( -32.45530648322815637, 41.13881078342074460, 2.056777965717148327 ) ) ;
#7725=CARTESIAN_POINT ( 'NONE',  ( -34.83316205860364079, 48.09832289792718285, -1.369967489524484883 ) ) ;
#7727=CARTESIAN_POINT ( 'NONE',  ( -31.30269415623623885, 33.99224428815358579, -1.031667027462585207 ) ) ;
#7728=LINE ( 'NONE', #2021, #11766 ) ;
#7737=CARTESIAN_POINT ( 'NONE',  ( -21.05849041552747281, 57.05917194494736577, 20.98221040122819403 ) ) ;
#7747=CARTESIAN_POINT ( 'NONE',  ( -34.22341864884656104, 49.42024689336786736, -4.283880285341411742 ) ) ;
#7749=VERTEX_POINT ( 'NONE', #4947 ) ;
#7753=CARTESIAN_POINT ( 'NONE',  ( 62.44550000000000267, 55.00000000000000000, 2.999999999999995559 ) ) ;
#7754=( GEOMETRIC_REPRESENTATION_CONTEXT ( 3 ) GLOBAL_UNCERTAINTY_ASSIGNED_CONTEXT ( ( #11289 ) ) GLOBAL_UNIT_ASSIGNED_CONTEXT ( ( #5611, #10140, #1038 ) ) REPRESENTATION_CONTEXT ( 'NONE', 'WORKASPACE' ) );
#7758=DIRECTION ( 'NONE',  ( -0.9999998346844721775, 0.0005712585774195265247, -6.553370117834432030E-05 ) ) ;
#7762=CARTESIAN_POINT ( 'NONE',  ( -24.47759590008010377, 52.25445690686086664, 21.01882782503509262 ) ) ;
#7764=CARTESIAN_POINT ( 'NONE',  ( -12.85572911067665380, 75.97954889423452585, -2.745668038893096519 ) ) ;
#7765=CARTESIAN_POINT ( 'NONE',  ( -42.66853512798572012, 55.00035148751268110, -14.01901578153819727 ) ) ;
#7770=CARTESIAN_POINT ( 'NONE',  ( -17.04105779988202585, 59.74509268894269098, 1.609841060220320141 ) ) ;
#7778=CARTESIAN_POINT ( 'NONE',  ( -21.12525410080779054, 58.60173025390926682, 6.007737297149077449 ) ) ;
#7780=CARTESIAN_POINT ( 'NONE',  ( -48.14429339001110009, 75.47411806927735256, -5.508782930744743567 ) ) ;
#7789=EDGE_LOOP ( 'NONE', ( #8488, #1909, #2297, #9453 ) ) ;
#7791=CARTESIAN_POINT ( 'NONE',  ( -78.00000000000000000, 54.99999999999999289, 0.000000000000000000 ) ) ;
#7793=CARTESIAN_POINT ( 'NONE',  ( -10.81092923698156838, 75.47407628921179423, -5.508885182882011122 ) ) ;
#7803=CARTESIAN_POINT ( 'NONE',  ( -50.87777401005003242, 59.84064543832867855, -1.293741243580276645 ) ) ;
#7806=CARTESIAN_POINT ( 'NONE',  ( -51.91627845054419765, 61.18957700299936420, 3.307427248076153070 ) ) ;
#7817=CARTESIAN_POINT ( 'NONE',  ( -14.83686862936316331, 54.99606387762347026, -0.004311921550151643669 ) ) ;
#7819=LINE ( 'NONE', #321, #310 ) ;
#7823=CARTESIAN_POINT ( 'NONE',  ( -46.39182477221876866, 68.38321102182860045, -16.29532114285349920 ) ) ;
#7826=CARTESIAN_POINT ( 'NONE',  ( 17.47768387407981905, 65.56544091938442875, 18.33174872895543928 ) ) ;
#7827=CARTESIAN_POINT ( 'NONE',  ( -8.544800298261920446, 62.20752307867830666, -12.02527808387988806 ) ) ;
#7828=PLANE ( 'NONE',  #9180 ) ;
#7830=CARTESIAN_POINT ( 'NONE',  ( -20.15075984075561522, 58.30274989043048350, 3.768099053302629731 ) ) ;
#7831=VECTOR ( 'NONE', #4849, 1000.000000000000000 ) ;
#7839=CARTESIAN_POINT ( 'NONE',  ( -51.55667834818763851, 61.98283010711340779, -0.9164068158849860701 ) ) ;
#7842=CARTESIAN_POINT ( 'NONE',  ( -55.50627899214600092, 66.73177265193905328, 17.54361557889675893 ) ) ;
#7843=CARTESIAN_POINT ( 'NONE',  ( 10.52240409369262153, 44.41989175727180594, 18.36819097564579195 ) ) ;
#7854=CARTESIAN_POINT ( 'NONE',  ( -13.85565285731654761, 75.43037139504293975, 5.490367781071763709 ) ) ;
#7868=CARTESIAN_POINT ( 'NONE',  ( -33.44321664797443105, 48.86004778347864885, -3.535033631877461335 ) ) ;
#7881=CARTESIAN_POINT ( 'NONE',  ( -9.759360353501660867, 55.02483400675389902, -0.008490801778254833052 ) ) ;
#7885=ORIENTED_EDGE ( 'NONE', *, *, #10019, .F. ) ;
#7887=CARTESIAN_POINT ( 'NONE',  ( -28.94161417925737823, 38.68453375511723635, 13.40299329694203578 ) ) ;
#7889=CARTESIAN_POINT ( 'NONE',  ( -61.78348097019890162, 49.89195498129476647, 20.38977643156359676 ) ) ;
#7890=CARTESIAN_POINT ( 'NONE',  ( -8.256150493756077680, 61.60926336870365105, -12.36828619365871695 ) ) ;
#7895=CARTESIAN_POINT ( 'NONE',  ( 11.81093755974026394, 42.10901286868706705, 16.77394813616862734 ) ) ;
#7899=CARTESIAN_POINT ( 'NONE',  ( 13.31285089744803862, 52.49279494320047235, 4.338208217070899764 ) ) ;
#7900=CARTESIAN_POINT ( 'NONE',  ( -35.41758684555698267, 48.28175916350203067, -2.038952528722552504 ) ) ;
#7902=CARTESIAN_POINT ( 'NONE',  ( -45.81092964171354964, 71.80742102382775727, -12.92463648794852205 ) ) ;
#7905=EDGE_CURVE ( 'NONE', #11420, #8851, #9966, .T. ) ;
#7913=CARTESIAN_POINT ( 'NONE',  ( -30.11869220662914159, 34.20731585996448132, 3.085050890631813036 ) ) ;
#7918=CARTESIAN_POINT ( 'NONE',  ( -30.36397657560652874, 35.99904827701746513, 8.986701095552454888 ) ) ;
#7923=CARTESIAN_POINT ( 'NONE',  ( 63.00000000000000000, 57.44550000000000267, 0.000000000000000000 ) ) ;
#7926=CARTESIAN_POINT ( 'NONE',  ( -58.04205566213050815, 55.34391004307462225, 6.992225127105330174 ) ) ;
#7937=CARTESIAN_POINT ( 'NONE',  ( 52.99999999999999289, 55.00000000000000000, -2.999999999999999112 ) ) ;
#7938=CARTESIAN_POINT ( 'NONE',  ( -19.49650547919373977, 55.00152523981414276, 0.004175815930542764627 ) ) ;
#7941=CARTESIAN_POINT ( 'NONE',  ( -28.67970331391730454, 50.16047344865108215, 1.298006186689315999 ) ) ;
#7942=CARTESIAN_POINT ( 'NONE',  ( -58.05785365788000263, 64.93276152744238061, 18.60033633024681521 ) ) ;
#7945=CARTESIAN_POINT ( 'NONE',  ( -53.33716864159804771, 74.42687709403668350, 8.047385144602918317 ) ) ;
#7946=CARTESIAN_POINT ( 'NONE',  ( -19.03633789442739399, 65.38143262936878841, 9.408964278925102676 ) ) ;
#7950=CARTESIAN_POINT ( 'NONE',  ( 5.451907626115248817, 34.19820075889870026, -3.085388827037094828 ) ) ;
#7953=DIRECTION ( 'NONE',  ( -1.000000000000000000, -6.033820786006286457E-17, -0.000000000000000000 ) ) ;
#7955=CARTESIAN_POINT ( 'NONE',  ( -31.04203254678103718, 48.66984814105956758, 2.994375663034408053 ) ) ;
#7957=CARTESIAN_POINT ( 'NONE',  ( 2.160190592651388908, 37.44772466133663613, -11.71846848753918913 ) ) ;
#7967=CARTESIAN_POINT ( 'NONE',  ( -3.608280849245335542, 57.05942974268126022, -21.01780866629736977 ) ) ;
#7970=AXIS2_PLACEMENT_3D ( 'NONE', #6977, #5058, #3134 ) ;
#7971=CARTESIAN_POINT ( 'NONE',  ( -67.97817662023267360, 50.66675960002082491, 2.515712352184921841 ) ) ;
#7973=CARTESIAN_POINT ( 'NONE',  ( -45.83980951013849392, 66.71822699054862937, -17.55167914569291554 ) ) ;
#7982=CARTESIAN_POINT ( 'NONE',  ( 25.33333333333333215, 69.00000000000001421, 0.000000000000000000 ) ) ;
#7993=CARTESIAN_POINT ( 'NONE',  ( -5.795201733763983398, 54.99589100033183087, 0.003790395536194273666 ) ) ;
#8003=CARTESIAN_POINT ( 'NONE',  ( -30.88142570102377604, 34.60150157552137529, 5.109735466913361890 ) ) ;
#8004=CARTESIAN_POINT ( 'NONE',  ( -54.33518187990853221, 67.95171888931189130, 5.365178638975860004 ) ) ;
#8011=DIRECTION ( 'NONE',  ( 0.000000000000000000, 0.000000000000000000, 1.000000000000000000 ) ) ;
#8014=CARTESIAN_POINT ( 'NONE',  ( 6.426141312414339168, 55.01574567783170977, -0.004739632326276670311 ) ) ;
#8015=ORIENTED_EDGE ( 'NONE', *, *, #6324, .T. ) ;
#8016=CARTESIAN_POINT ( 'NONE',  ( -10.05849041713385716, 73.59815716747449699, -9.932440597164658769 ) ) ;
#8024=CARTESIAN_POINT ( 'NONE',  ( 53.00000000000000000, 51.46446609406726935, -3.535533905932738197 ) ) ;
#8026=CARTESIAN_POINT ( 'NONE',  ( -57.82750524721426189, 59.10997802641301035, 20.69196764327204008 ) ) ;
#8041=CARTESIAN_POINT ( 'NONE',  ( 4.378415270005670656, 50.50465253094520790, -2.213690094899597227 ) ) ;
#8042=CARTESIAN_POINT ( 'NONE',  ( -22.87290721160892559, 51.34344131888308738, 13.61233213364711858 ) ) ;
#8050=EDGE_CURVE ( 'NONE', #3861, #1195, #496, .T. ) ;
#8054=CARTESIAN_POINT ( 'NONE',  ( -10.57393008609709284, 54.97382464119526446, -0.001646660502260763022 ) ) ;
#8059=CARTESIAN_POINT ( 'NONE',  ( -16.62112305147868341, 58.30599534545817875, 3.765284532852771537 ) ) ;
#8063=CARTESIAN_POINT ( 'NONE',  ( -58.60805698665915742, 61.13948054013681599, 20.20364628154455033 ) ) ;
#8067=ADVANCED_FACE ( 'NONE', ( #616, #5243 ), #9665, .T. ) ;
#8070=ORIENTED_EDGE ( 'NONE', *, *, #10002, .F. ) ;
#8073=CARTESIAN_POINT ( 'NONE',  ( 19.52230480204648799, 67.92440004991483704, 16.80766691833610693 ) ) ;
#8077=CARTESIAN_POINT ( 'NONE',  ( 12.53471759186635914, 51.95107372724174155, 3.976201241736514902 ) ) ;
#8079=CARTESIAN_POINT ( 'NONE',  ( -63.41718291383947559, 52.96799456708508558, 6.699226218324908722 ) ) ;
#8082=CARTESIAN_POINT ( 'NONE',  ( -60.45014771802851072, 49.89223742090062075, 20.38901927491476584 ) ) ;
#8083=CARTESIAN_POINT ( 'NONE',  ( -20.45202553191040806, 65.80759480864719535, 18.03021102644938267 ) ) ;
#8091=CARTESIAN_POINT ( 'NONE',  ( -39.16026728571524984, 50.89059911655681390, -20.69167526169209026 ) ) ;
#8100=ORIENTED_EDGE ( 'NONE', *, *, #5718, .T. ) ;
#8102=ORIENTED_EDGE ( 'NONE', *, *, #6324, .F. ) ;
#8103=CARTESIAN_POINT ( 'NONE',  ( 2.818321079511319827, 51.23034582308294915, -3.301094900672958410 ) ) ;
#8104=CARTESIAN_POINT ( 'NONE',  ( -1.872832575621271589, 53.16883357371531105, -13.97545723436864762 ) ) ;
#8109=VERTEX_POINT ( 'NONE', #6030 ) ;
#8114=CARTESIAN_POINT ( 'NONE',  ( -30.28557338859272718, 54.99143721797869944, -0.0008624110448812779411 ) ) ;
#8121=CARTESIAN_POINT ( 'NONE',  ( -59.16083848046626059, 59.10996271935812274, 20.69255083878625712 ) ) ;
#8125=CARTESIAN_POINT ( 'NONE',  ( -13.14429486149114013, 76.02373996650987920, 2.745652855075435994 ) ) ;
#8128=CARTESIAN_POINT ( 'NONE',  ( 16.57387832582033838, 55.01040436726604810, 0.01274895920632791203 ) ) ;
#8130=CARTESIAN_POINT ( 'NONE',  ( -4.826933883979098283, 59.12189523993642126, -20.68950996840993284 ) ) ;
#8131=CARTESIAN_POINT ( 'NONE',  ( -9.070746587277097817, 68.33487957594263662, -16.24597445391072270 ) ) ;
#8143=CARTESIAN_POINT ( 'NONE',  ( -62.53961969342599048, 54.34518536178778447, 4.967644874103720909 ) ) ;
#8146=CARTESIAN_POINT ( 'NONE',  ( 36.99999999999999289, 50.00000000000001421, 6.123233995736750505E-16 ) ) ;
#8148=CARTESIAN_POINT ( 'NONE',  ( 21.45655948015391701, 59.96735746368497644, 0.6566347522681182936 ) ) ;
#8156=CARTESIAN_POINT ( 'NONE',  ( 2.595294705192281892, 44.14252394839951421, -8.915488700345314044 ) ) ;
#8166=CARTESIAN_POINT ( 'NONE',  ( -15.09523335307150838, 60.00000000000000000, 4.640896189903090912E-12 ) ) ;
#8168=CARTESIAN_POINT ( 'NONE',  ( -56.83651104956651778, 55.00013208380096330, -0.005320426939399679200 ) ) ;
#8172=CARTESIAN_POINT ( 'NONE',  ( -19.34581284733777551, 56.29866528490898503, 4.839339984244626081 ) ) ;
#8177=CARTESIAN_POINT ( 'NONE',  ( 16.81101720596863203, 65.56606704192360269, 18.33326034385300574 ) ) ;
#8184=CARTESIAN_POINT ( 'NONE',  ( -3.608280849245335542, 57.05942974268126022, -21.01780866629736977 ) ) ;
#8187=CARTESIAN_POINT ( 'NONE',  ( 5.097072204971999199, 54.98817743756426779, 0.003549163818565345425 ) ) ;
#8190=CARTESIAN_POINT ( 'NONE',  ( -66.81799029952708224, 34.52069382205590387, 5.503409927558503334 ) ) ;
#8191=CARTESIAN_POINT ( 'NONE',  ( -27.52231952827322559, 42.10572610250680015, 16.77759997522909785 ) ) ;
#8199=CARTESIAN_POINT ( 'NONE',  ( -51.09272475326343965, 55.01575874039146896, -0.004732945744491365812 ) ) ;
#8200=CARTESIAN_POINT ( 'NONE',  ( -46.38003273829423279, 59.55718620543969877, -2.063744646361077795 ) ) ;
#8201=FACE_OUTER_BOUND ( 'NONE', #2029, .T. ) ;
#8202=CARTESIAN_POINT ( 'NONE',  ( -57.48338928910774825, 58.30336033756839953, 3.767575935608591386 ) ) ;
#8204=DIRECTION ( 'NONE',  ( 1.000000000000000000, 6.033820786006286457E-17, -0.000000000000000000 ) ) ;
#8206=CARTESIAN_POINT ( 'NONE',  ( 14.84754529999163175, 56.60743895240869961, 4.745939591966136462 ) ) ;
#8214=CARTESIAN_POINT ( 'NONE',  ( -7.676230545052211696, 58.97267896026763623, -3.053804416834208890 ) ) ;
#8216=CARTESIAN_POINT ( 'NONE',  ( -18.41060825077335394, 61.60246496029746766, 12.35359534585878549 ) ) ;
#8219=DIRECTION ( 'NONE',  ( -0.04756514941544910668, -0.9988681377244376103, 0.000000000000000000 ) ) ;
#8227=CARTESIAN_POINT ( 'NONE',  ( -49.83687785813567928, 54.99470118834590693, -0.002487210696061862344 ) ) ;
#8231=CARTESIAN_POINT ( 'NONE',  ( -12.35069320478294230, 59.96772244320774092, 0.6536033618355622243 ) ) ;
#8235=CARTESIAN_POINT ( 'NONE',  ( -17.82693376281896391, 72.53768310958322729, 11.72612467905221934 ) ) ;
#8240=CARTESIAN_POINT ( 'NONE',  ( -34.14426257084027583, 36.62727174719971401, -10.58198811264723282 ) ) ;
#8242=ORIENTED_EDGE ( 'NONE', *, *, #11792, .T. ) ;
#8245=CARTESIAN_POINT ( 'NONE',  ( -70.22791978040648075, 48.01650020567630150, 0.9109789678819780745 ) ) ;
#8247=CARTESIAN_POINT ( 'NONE',  ( -32.83980940775745694, 34.29934832242292231, -4.109488215307584014 ) ) ;
#8249=CARTESIAN_POINT ( 'NONE',  ( -10.83980928483403794, 72.54296691076741865, -11.73126556815853760 ) ) ;
#8250=FACE_OUTER_BOUND ( 'NONE', #6178, .T. ) ;
#8251=FACE_OUTER_BOUND ( 'NONE', #11349, .T. ) ;
#8254=EDGE_CURVE ( 'NONE', #1114, #3047, #7224, .T. ) ;
#8256=CARTESIAN_POINT ( 'NONE',  ( -45.95223880245733028, 55.00272212807455929, -0.004616914605015018727 ) ) ;
#8257=CARTESIAN_POINT ( 'NONE',  ( -43.46451671436751241, 58.04975000076846925, -3.975644651036446486 ) ) ;
#8264=CARTESIAN_POINT ( 'NONE',  ( -33.76207074264209496, 50.00000000000002842, -7.785926851161516095E-15 ) ) ;
#8265=CARTESIAN_POINT ( 'NONE',  ( 11.34649352705233305, 53.70496425952375574, 4.840325120478907728 ) ) ;
#8272=CARTESIAN_POINT ( 'NONE',  ( -1.847600398352776008, 54.66814614765320357, -4.991699084503711248 ) ) ;
#8273=CARTESIAN_POINT ( 'NONE',  ( -16.66853507982470717, 64.91323907223390677, 9.913723736632611860 ) ) ;
#8281=EDGE_CURVE ( 'NONE', #443, #5990, #3278, .T. ) ;
#8282=CARTESIAN_POINT ( 'NONE',  ( -47.90718171337187670, 54.97383743986804916, -0.001639851572109073119 ) ) ;
#8289=DIRECTION ( 'NONE',  ( 0.000000000000000000, 1.000000000000000000, 0.000000000000000000 ) ) ;
#8292=CARTESIAN_POINT ( 'NONE',  ( 0.2748429140369315071, 38.70467982241823535, -13.38321124372595783 ) ) ;
#8296=CARTESIAN_POINT ( 'NONE',  ( -19.63602748969081446, 62.08618401115764129, 19.80343740535094099 ) ) ;
#8299=AXIS2_PLACEMENT_3D ( 'NONE', #6649, #2077, #5751 ) ;
#8300=CARTESIAN_POINT ( 'NONE',  ( -11.98451233991428744, 59.33800141420930885, -2.507694870718707225 ) ) ;
#8301=CARTESIAN_POINT ( 'NONE',  ( 3.737309610555803463, 34.06887424008940712, -2.059134394038261817 ) ) ;
#8303=CARTESIAN_POINT ( 'NONE',  ( -54.11877253047997982, 71.88441139826683468, 12.52138966593202341 ) ) ;
#8304=CARTESIAN_POINT ( 'NONE',  ( -44.96936008568403764, 63.99178041037959019, -19.01235157881157178 ) ) ;
#8310=CARTESIAN_POINT ( 'NONE',  ( -21.75699517953123774, 54.99788995967445970, -0.006179814837821989357 ) ) ;
#8311=CARTESIAN_POINT ( 'NONE',  ( -52.79756777621546604, 58.97512417236831794, 3.050472611213659313 ) ) ;
#8312=CARTESIAN_POINT ( 'NONE',  ( 25.00000000000000000, 76.00000000000000000, 0.000000000000000000 ) ) ;
#8314=CARTESIAN_POINT ( 'NONE',  ( -2.556751989345197984, 51.48122000982115765, -6.100625743585796457 ) ) ;
#8316=CARTESIAN_POINT ( 'NONE',  ( 14.85570562722353749, 52.25434861561973321, 21.02374011750137939 ) ) ;
#8327=CARTESIAN_POINT ( 'NONE',  ( -42.33147328884727045, 60.36255737924431486, -12.94746809434214541 ) ) ;
#8337=CARTESIAN_POINT ( 'NONE',  ( -59.46281197144560338, 55.00344839445808276, -0.006247678623671736216 ) ) ;
#8341=FACE_OUTER_BOUND ( 'NONE', #5684, .T. ) ;
#8347=ORIENTED_EDGE ( 'NONE', *, *, #9461, .F. ) ;
#8348=CARTESIAN_POINT ( 'NONE',  ( 2.003855453843550460, 35.57695044197526357, -8.044733130177707636 ) ) ;
#8352=CARTESIAN_POINT ( 'NONE',  ( -34.85572910849313644, 38.22605186251247744, -12.89098713163435228 ) ) ;
#8357=CARTESIAN_POINT ( 'NONE',  ( -65.17448922114576249, 36.67438677247554324, 10.54995967583099237 ) ) ;
#8360=CARTESIAN_POINT ( 'NONE',  ( -2.651582617587235458, 52.49162778365467830, -4.337637646355388732 ) ) ;
#8363=CARTESIAN_POINT ( 'NONE',  ( -23.85572910907371025, 49.50876680309251299, 20.43178602932799492 ) ) ;
#8364=AXIS2_PLACEMENT_3D ( 'NONE', #6568, #8473, #8528 ) ;
#8365=CARTESIAN_POINT ( 'NONE',  ( -66.47562283042974229, 38.19906477560226676, 12.92409071120044040 ) ) ;
#8374=CARTESIAN_POINT ( 'NONE',  ( -23.49650511202184688, 55.00077215910898332, 0.002398592362466134536 ) ) ;
#8375=CARTESIAN_POINT ( 'NONE',  ( -42.68304982271171610, 57.50651106462216688, -4.338678109911903391 ) ) ;
#8378=CARTESIAN_POINT ( 'NONE',  ( 1.333197741078869125, 48.52671685189832829, -2.680978973290799150 ) ) ;
#8380=CARTESIAN_POINT ( 'NONE',  ( 24.18742635297404675, 76.02379904146428657, 2.751050496637376774 ) ) ;
#8393=CARTESIAN_POINT ( 'NONE',  ( -62.17173789034691112, 47.18625706333304493, 11.70555309606978689 ) ) ;
#8400=CARTESIAN_POINT ( 'NONE',  ( -34.73940033462148591, 50.06485160516485422, -0.8190406228260763699 ) ) ;
#8403=CARTESIAN_POINT ( 'NONE',  ( -6.417135814581119035, 59.43955965505210060, -5.410182326209246106 ) ) ;
#8408=CARTESIAN_POINT ( 'NONE',  ( 62.44550000000000267, 55.00000000000000000, 0.000000000000000000 ) ) ;
#8412=CARTESIAN_POINT ( 'NONE',  ( -68.86034823945129801, 34.02049636744572325, 2.749403782478469616 ) ) ;
#8417=CARTESIAN_POINT ( 'NONE',  ( -52.59603425219209782, 73.55155261293346314, 9.913157997185967574 ) ) ;
#8418=SURFACE_STYLE_FILL_AREA ( #10205 ) ;
#8419=CARTESIAN_POINT ( 'NONE',  ( -53.45210586504737904, 71.88419113761085555, 12.52116934359859002 ) ) ;
#8422=CARTESIAN_POINT ( 'NONE',  ( -11.20418418299178320, 58.97469996104722156, -3.050991650916503595 ) ) ;
#8426=CARTESIAN_POINT ( 'NONE',  ( -33.39182374990940616, 34.82582084984149873, -6.127586950986167125 ) ) ;
#8427=CARTESIAN_POINT ( 'NONE',  ( -52.82691659388441252, 75.69008924411679118, 4.122156975067814422 ) ) ;
#8434=CARTESIAN_POINT ( 'NONE',  ( -16.09272391817585657, 55.01637097774587204, 0.001658295702028558935 ) ) ;
#8435=CARTESIAN_POINT ( 'NONE',  ( -48.12550986829561595, 59.96676360895955327, -0.6610507428945817665 ) ) ;
#8443=CARTESIAN_POINT ( 'NONE',  ( -1.776549974196238946, 50.68601013462039617, -5.609814685327735972 ) ) ;
#8458=CARTESIAN_POINT ( 'NONE',  ( -47.79377051319855241, 68.65769002727881798, -3.675352279733770544 ) ) ;
#8469=CARTESIAN_POINT ( 'NONE',  ( -18.08380248123574319, 58.29941079146190930, 6.172005441165978823 ) ) ;
#8470=CARTESIAN_POINT ( 'NONE',  ( 62.44550000000000267, 55.00000000000000000, -2.999999999999995559 ) ) ;
#8473=DIRECTION ( 'NONE',  ( 1.000000000000000000, 6.033820786006286457E-17, -0.000000000000000000 ) ) ;
#8477=CARTESIAN_POINT ( 'NONE',  ( -43.21475900837984341, 58.08538667521604282, -20.80084980650556759 ) ) ;
#8480=CARTESIAN_POINT ( 'NONE',  ( -50.27495406422890767, 76.01781437481966464, 2.059423474151367728 ) ) ;
#8486=CARTESIAN_POINT ( 'NONE',  ( -9.656863044840665822, 58.05255974435234378, -3.973617159649989183 ) ) ;
#8487=CARTESIAN_POINT ( 'NONE',  ( 17.52230480588388417, 67.92092721363508190, 16.80419350660125843 ) ) ;
#8488=ORIENTED_EDGE ( 'NONE', *, *, #6057, .T. ) ;
#8489=CARTESIAN_POINT ( 'NONE',  ( -21.72515708326280048, 57.05917195472675019, 20.98343720861656436 ) ) ;
#8490=CARTESIAN_POINT ( 'NONE',  ( -63.63584090060282961, 46.00639722032484968, 19.01118640546643590 ) ) ;
#8494=CARTESIAN_POINT ( 'NONE',  ( 36.99999999999999289, 55.00000000000000000, 0.000000000000000000 ) ) ;
#8497=CARTESIAN_POINT ( 'NONE',  ( -67.42686117391447453, 54.98684645604348020, 0.008483758310626438731 ) ) ;
#8500=CARTESIAN_POINT ( 'NONE',  ( 3.666806354490720565, 47.98949887324683061, -0.0002676899127992829822 ) ) ;
#8502=CARTESIAN_POINT ( 'NONE',  ( -5.337209886265139147, 63.04750289227570192, -19.42727033598380970 ) ) ;
#8505=DIRECTION ( 'NONE',  ( -0.000000000000000000, -0.000000000000000000, 1.000000000000000000 ) ) ;
#8506=CARTESIAN_POINT ( 'NONE',  ( 4.350743830703725834, 50.03278576500255070, 0.6577445178750861432 ) ) ;
#8513=CARTESIAN_POINT ( 'NONE',  ( 24.18742635297404675, 76.02379904146428657, 2.751050496637376774 ) ) ;
#8522=FACE_OUTER_BOUND ( 'NONE', #5379, .T. ) ;
#8524=CARTESIAN_POINT ( 'NONE',  ( -17.20817491345679784, 59.17780944700501777, 5.632517163406045135 ) ) ;
#8528=DIRECTION ( 'NONE',  ( 0.000000000000000000, 1.000000000000000000, 0.000000000000000000 ) ) ;
#8532=CARTESIAN_POINT ( 'NONE',  ( -61.88037028687247698, 51.91449295574040690, 20.80032498971814192 ) ) ;
#8541=CARTESIAN_POINT ( 'NONE',  ( 53.00000000000004974, 4.648349522099639420E-14, 0.000000000000000000 ) ) ;
#8542=CARTESIAN_POINT ( 'NONE',  ( 22.18771278451687579, 76.01886845420673922, 2.750080521686579793 ) ) ;
#8545=CARTESIAN_POINT ( 'NONE',  ( -60.54703689898057206, 51.91451759569049784, 20.80086399049218215 ) ) ;
#8546=CARTESIAN_POINT ( 'NONE',  ( -53.69727390230763575, 74.79022971164903311, 7.081167078663678893 ) ) ;
#8548=CARTESIAN_POINT ( 'NONE',  ( 53.00000000000000000, 51.46446609406726935, 3.535533905932731091 ) ) ;
#8556=LINE ( 'NONE', #8312, #9921 ) ;
#8559=CARTESIAN_POINT ( 'NONE',  ( -4.890012301214623491, 54.08359342507363721, -6.982820483012029733 ) ) ;
#8562=CARTESIAN_POINT ( 'NONE',  ( -17.59602449223222109, 68.34579465778965357, 16.25793134507749826 ) ) ;
#8569=ORIENTED_EDGE ( 'NONE', *, *, #9953, .F. ) ;
#8574=AXIS2_PLACEMENT_3D ( 'NONE', #3677, #11752, #2727 ) ;
#8575=CARTESIAN_POINT ( 'NONE',  ( -57.49717384800269571, 57.74002937887566844, 13.79287161986824017 ) ) ;
#8590=CARTESIAN_POINT ( 'NONE',  ( 21.77666841074465864, 60.57982234150205869, 4.283804165148911380 ) ) ;
#8600=CARTESIAN_POINT ( 'NONE',  ( -57.50627882723209439, 66.73110044028416610, 17.54296274220338958 ) ) ;
#8603=DIRECTION ( 'NONE',  ( -0.04699449999129696326, 0.9988950444178830157, -0.0004552010143329844735 ) ) ;
#8609=CARTESIAN_POINT ( 'NONE',  ( -8.785358865379802040, 67.52185545713140868, -16.88477868139494831 ) ) ;
#8610=ORIENTED_EDGE ( 'NONE', *, *, #4766, .T. ) ;
#8611=CARTESIAN_POINT ( 'NONE',  ( 19.81102887321632622, 71.77647403800290249, 12.89307786291128899 ) ) ;
#8612=VECTOR ( 'NONE', #5922, 1000.000000000000000 ) ;
#8613=CARTESIAN_POINT ( 'NONE',  ( 1.668526597461617023, 42.05183364693759529, -5.362856051735069407 ) ) ;
#8621=CARTESIAN_POINT ( 'NONE',  ( -19.37536588012664041, 60.18888662840161885, 4.702399783581789450 ) ) ;
#8623=CARTESIAN_POINT ( 'NONE',  ( -52.88146049032556562, 73.03766007303350705, 10.81102556547625149 ) ) ;
#8625=LINE ( 'NONE', #5036, #5634 ) ;
#8634=CARTESIAN_POINT ( 'NONE',  ( -7.969360823174009845, 70.58422527244209732, -14.12522777056770629 ) ) ;
#8645=CARTESIAN_POINT ( 'NONE',  ( -40.37827046521217511, 52.78600536084015715, -4.495190126649539764 ) ) ;
#8647=CARTESIAN_POINT ( 'NONE',  ( -10.10988331466380430, 61.84124810089927138, -1.841955595480224250 ) ) ;
#8654=EDGE_LOOP ( 'NONE', ( #5421, #9148, #4267, #1413 ) ) ;
#8655=CARTESIAN_POINT ( 'NONE',  ( -61.59556246352555320, 52.94114603458827872, 20.93095456750423722 ) ) ;
#8656=B_SPLINE_CURVE_WITH_KNOTS ( 'NONE', 3,
 ( #9441, #4110, #6644, #10276, #7770, #11399, #3213, #1230, #4898, #7830, #6943, #2370, #11462, #6043, #9680, #10569, #3270, #5081, #8726, #507, #4170, #6540, #10997, #6414, #1904, #2022, #9991, #1966, #2809, #8264 ),
 .UNSPECIFIED., .F., .F.,
 ( 4, 2, 2, 2, 2, 2, 2, 2, 2, 2, 2, 2, 2, 2, 4 ),
 ( 0.04856964348838239964, 0.05008746542464584395, 0.05160528736090929519, 0.05312310929717274643, 0.05464093123343619074, 0.05615875316969964198, 0.05767657510596308629, 0.06071221897849000265, 0.06223004091475346777, 0.06374786285101693983, 0.06526568478728039802, 0.06678350672354385620, 0.06830132865980732826, 0.06981915059607078644, 0.07285479446859771668 ),
 .UNSPECIFIED. ) ;
#8658=ADVANCED_FACE ( 'NONE', ( #4692 ), #7520, .T. ) ;
#8660=LINE ( 'NONE', #9489, #2407 ) ;
#8665=ADVANCED_FACE ( 'NONE', ( #5839 ), #10825, .T. ) ;
#8666=CARTESIAN_POINT ( 'NONE',  ( -22.50647595179652072, 59.12487335784310005, 20.69694904210189179 ) ) ;
#8668=CARTESIAN_POINT ( 'NONE',  ( -17.16026715680585824, 72.53745844446059721, 11.72589600754185035 ) ) ;
#8669=CARTESIAN_POINT ( 'NONE',  ( -19.92281716047341433, 63.89755087529745481, 10.83930136440029202 ) ) ;
#8670=CARTESIAN_POINT ( 'NONE',  ( 37.00000000000000000, 55.00000000000000000, 0.000000000000000000 ) ) ;
#8671=DIRECTION ( 'NONE',  ( 1.000000000000000000, 6.033820786006286457E-17, -0.000000000000000000 ) ) ;
#8675=CARTESIAN_POINT ( 'NONE',  ( -68.34104732181945963, 33.99448141944315438, 0.006743540747239065887 ) ) ;
#8678=CARTESIAN_POINT ( 'NONE',  ( -43.87484156505298216, 56.02863006267562440, -6.935366095584925006 ) ) ;
#8680=CARTESIAN_POINT ( 'NONE',  ( -17.88142570751413274, 67.52739394234649239, 16.89079266652326439 ) ) ;
#8681=CARTESIAN_POINT ( 'NONE',  ( 23.00000000000000000, 76.00000000000000000, 0.000000000000000000 ) ) ;
#8691=CARTESIAN_POINT ( 'NONE',  ( -28.36397722366938012, 36.00052710555507218, 8.986026874162561739 ) ) ;
#8694=DIRECTION ( 'NONE',  ( 1.000000000000000000, 6.033820786006286457E-17, 0.000000000000000000 ) ) ;
#8701=CARTESIAN_POINT ( 'NONE',  ( -44.07273810123712110, 55.81934495312422939, -4.935102682546041564 ) ) ;
#8703=CARTESIAN_POINT ( 'NONE',  ( -42.29128031504409080, 58.00020108910005234, -6.342998449018511842 ) ) ;
#8712=ADVANCED_FACE ( 'NONE', ( #8341 ), #9419, .T. ) ;
#8714=CARTESIAN_POINT ( 'NONE',  ( -8.430468385592622127, 54.98139370647056978, 0.006371973333601899971 ) ) ;
#8718=CARTESIAN_POINT ( 'NONE',  ( -32.11869219899978845, 34.20636958863568822, 3.085052597841025701 ) ) ;
#8720=CARTESIAN_POINT ( 'NONE',  ( -8.118692201255964136, 67.52163282122538135, -16.88455524069670233 ) ) ;
#8721=CARTESIAN_POINT ( 'NONE',  ( -38.79377121134427142, 46.38247438902519093, -11.20693327228071468 ) ) ;
#8724=B_SPLINE_SURFACE_WITH_KNOTS ( 'NONE', 3, 3, ( 
 ( #11174, #8380, #5695, #3945, #7369, #5569, #2808, #4607, #6598, #8316, #226, #6655, #9216, #10289, #161, #3831, #3889, #1004, #2869, #2083, #7496, #10103, #6536, #5757, #7609, #10168, #2020, #9269, #9394, #38, #9332, #4788, #1188, #4853, #8502, #1122, #4663, #3048, #1901, #6718, #10350, #5510, #941, #11531, #4070, #10460, #6835, #5145, #1240, #5034, #9631, #8562, #8680, #5933, #3281, #11412, #4972, #10518, #2325, #6778, #2147, #11302, #10405, #2378, #405, #1426, #342, #9574, #1371, #10577, #463, #8798, #7727, #6951, #5997, #11358, #4910, #576, #3112, #2261, #4120, #6053, #7667, #9688, #9455, #4008, #5817, #2205, #1486, #5872, #4243, #7902, #3337, #7780, #5089, #7007, #3165, #3222, #6891, #8736, #8623, #9514, #1304, #519, #4181, #7842, #11470, #1540, #1652, #9918, #7246, #3575, #1771, #8082, #10696, #692, #636, #11715, #2618, #6171, #2681, #8190, #4365, #7130 ),
 ( #4534, #11655, #11826, #4298, #863, #4424, #2444, #3515, #3633, #6110, #10809, #809, #6228, #4478, #7184, #5207, #10868, #9743, #9802, #6345, #5437, #750, #10629, #8857, #1716, #7957, #11591, #9976, #6287, #5380, #3397, #9084, #8130, #3464, #7070, #2506, #2561, #9032, #1596, #11768, #5264, #8911, #8016, #10752, #9859, #5321, #8974, #5677, #6400, #10148, #11158, #1106, #2741, #1949, #7414, #2973, #2917, #5618, #8489, #84, #8363, #7356, #9198, #2793, #10212, #10030, #1884, #3692, #10271, #3747, #1823, #6639, #2069, #8247, #8426, #145, #5492, #9317, #9257, #7481, #5740, #9142, #10981, #923, #4591, #1047, #10087, #2005, #4770, #6457, #989, #24, #4712, #11102, #5555, #9376, #4837, #4650, #11042, #2850, #1169, #8303, #3811, #6582, #6520, #210, #3875, #7536, #267, #7301, #10931, #449, #8545, #3930, #1226, #327, #4165, #2187, #11395, #10333, #7714, #11343, #503, #3151 ),
 ( #5859, #6702, #2367, #4893, #8611, #389, #7826, #9437, #5077, #11223, #2130, #7594, #3992, #11458, #5803, #7652, #1414, #11285, #3098, #9498, #10504, #3267, #2308, #5021, #6938, #1354, #10566, #9560, #1288, #6764, #10391, #4955, #5985, #6039, #3033, #9675, #1471, #8720, #4058, #6819, #5134, #4106, #10445, #9619, #7764, #8782, #2247, #5916, #8668, #3209, #6877, #3326, #2491, #7234, #5192, #1703, #8899, #8963, #10796, #679, #10617, #6155, #6994, #2428, #4352, #10859, #3562, #11756, #8003, #737, #9963, #9791, #11638, #3444, #4412, #3381, #9019, #2667, #7058, #6214, #10678, #7172, #6096, #7116, #11705, #795, #5367, #6334, #9847, #623, #9728, #4287, #1528, #11520, #1639, #1584, #3505, #6276, #7945, #9907, #10741, #2548, #2607, #11579, #5252, #4469, #5308, #8063, #8121, #1759, #5424, #563, #4230, #7889, #8844, #1034, #70, #7467, #3621, #3734, #194, #10073, #8412, #7400 ),
 ( #1095, #6628, #10970, #5539, #1872, #3863, #8177, #11028, #4697, #7288, #2837, #975, #10200, #6505, #12, #5607, #9246, #1811, #9074, #6388, #5479, #9301, #7345, #8348, #10919, #4640, #8292, #5664, #10133, #7525, #2781, #1994, #132, #6443, #11816, #11147, #10016, #9186, #1935, #4759, #2731, #2962, #4522, #9128, #850, #909, #10258, #4580, #8235, #6572, #3682, #3797, #11090, #2903, #2055, #4260, #6805, #1559, #3139, #9760, #11331, #11270, #3021, #2115, #9425, #7918, #5225, #5729, #6126, #652, #10648, #6688, #7640, #3352, #2235, #7583, #11549, #5904, #2459, #9485, #8873, #3981, #1154, #435, #8477, #3081, #4317, #10319, #7025, #7973, #11610, #10433, #5792, #6752, #11210, #9548, #1343, #1215, #3413, #7087, #10380, #2175, #5844, #10711, #4824, #8600, #5006, #253, #376, #1275, #9363, #8655, #8532, #3918, #4881, #316, #4943, #4041, #7698, #2756, #767, #9992, #8930, #6304 ) ),
 .UNSPECIFIED., .F., .F., .F.,
 ( 4, 4 ),
 ( 4, 2, 2, 2, 2, 2, 2, 2, 2, 2, 2, 2, 2, 2, 2, 2, 2, 2, 2, 2, 2, 2, 2, 2, 2, 2, 2, 2, 2, 2, 2, 2, 2, 2, 2, 2, 2, 2, 2, 2, 2, 2, 2, 2, 2, 2, 2, 2, 2, 2, 2, 2, 2, 2, 2, 2, 2, 2, 2, 2, 2, 4 ),
 ( 0.000000000000000000, 1.000000000000000000 ),
 ( 0.000000000000000000, 0.02499977550252127645, 0.04999988577693819519, 0.07499999605135511394, 0.09999999831535408279, 0.1250000005793530378, 0.1500000028441162425, 0.1750000051088794195, 0.1937500039558066045, 0.2031250033792701970, 0.2125000028027338173, 0.2218750022261974375, 0.2312500016496610300, 0.2500000004965882150, 0.2750000027613288545, 0.3000000050260694384, 0.3187500038730080032, 0.3281250032964772578, 0.3375000027199465125, 0.3468750021434158226, 0.3562500015668850772, 0.3750000004138236420, 0.4000000026785641705, 0.4250000049433046989, 0.4437500037902432082, 0.4531250032137125183, 0.4625000026371817730, 0.4718750020606510276, 0.4812500014841203377, 0.5000000003310588470, 0.5250000025957997085, 0.5500000048605405700, 0.5687500037074788573, 0.5781250031309480564, 0.5875000025544172555, 0.5968750019778864546, 0.6062500014013556537, 0.6250000002482940520, 0.6500000025128280789, 0.6750000047773621059, 0.6937500036244039769, 0.7031250030479249125, 0.7125000024714458480, 0.7218750018949667835, 0.7312500013184877190, 0.7500000001655295900, 0.7750000023794885173, 0.8000000045934475557, 0.8187500034657768655, 0.8281250029019414649, 0.8375000023381060643, 0.8468750017742707747, 0.8562500012104353742, 0.8750000000827646840, 0.8937502654913498379, 0.9031253981956424148, 0.9125005308999349918, 0.9218756636042275687, 0.9312507963085201457, 0.9500010617171052996, 0.9750005308585526498, 1.000000000000000000 ),
 .UNSPECIFIED. ) ;
#8726=CARTESIAN_POINT ( 'NONE',  ( -26.37503197251934850, 53.38964644461982090, 4.744911376643659473 ) ) ;
#8733=CARTESIAN_POINT ( 'NONE',  ( -20.54150823158944661, 59.17669310859397314, 5.631395700702261919 ) ) ;
#8736=CARTESIAN_POINT ( 'NONE',  ( -52.59603425219209782, 73.55155261293346314, 9.913157997185967574 ) ) ;
#8747=CARTESIAN_POINT ( 'NONE',  ( 9.477680475861957277, 36.67126955513442255, 10.56417786655960356 ) ) ;
#8753=ORIENTED_EDGE ( 'NONE', *, *, #11425, .F. ) ;
#8762=CARTESIAN_POINT ( 'NONE',  ( -53.66679727893465923, 59.95398294780274995, 4.953507936222676378 ) ) ;
#8775=CARTESIAN_POINT ( 'NONE',  ( -4.909738907900197624, 55.00455243144571682, -0.008585322715572331689 ) ) ;
#8777=ORIENTED_EDGE ( 'NONE', *, *, #8281, .T. ) ;
#8780=CARTESIAN_POINT ( 'NONE',  ( -48.52239103406665066, 73.33336493528216238, -10.56581381373428208 ) ) ;
#8782=CARTESIAN_POINT ( 'NONE',  ( -14.47762819197135364, 76.02046563874422702, 2.745652569741364957 ) ) ;
#8783=CARTESIAN_POINT ( 'NONE',  ( -22.83648567187163181, 57.75017295826287977, 13.79876555885540590 ) ) ;
#8794=CARTESIAN_POINT ( 'NONE',  ( 9.042618572576390790, 50.25505735147245190, 1.610274559975814812 ) ) ;
#8795=CARTESIAN_POINT ( 'NONE',  ( -31.33319364550761321, 48.52303905584467003, 2.682555320553783762 ) ) ;
#8796=AXIS2_PLACEMENT_3D ( 'NONE', #8024, #6295, #7253 ) ;
#8798=CARTESIAN_POINT ( 'NONE',  ( -30.99614452189004155, 33.97742542711323921, 0.0005215828242728561687 ) ) ;
#8811=CARTESIAN_POINT ( 'NONE',  ( -9.391823749396904120, 73.59702374900430755, -9.931971109272440756 ) ) ;
#8813=EDGE_CURVE ( 'NONE', #3881, #3861, #11781, .T. ) ;
#8822=PRODUCT_DEFINITION_CONTEXT ( 'detailed design', #11501, 'design' ) ;
#8823=ORIENTED_EDGE ( 'NONE', *, *, #2725, .T. ) ;
#8824=CARTESIAN_POINT ( 'NONE',  ( -67.66638273083707134, 47.99409686189664370, 0.0004508834932907918535 ) ) ;
#8836=CARTESIAN_POINT ( 'NONE',  ( 24.42601517758169294, 54.97644996077841739, -0.01153606584382102333 ) ) ;
#8841=CARTESIAN_POINT ( 'NONE',  ( -29.84797894700232490, 49.99999999999998579, 0.3308608129958152677 ) ) ;
#8842=CARTESIAN_POINT ( 'NONE',  ( -30.67054324275970600, 35.57292846186890500, 8.046485333435041909 ) ) ;
#8844=CARTESIAN_POINT ( 'NONE',  ( -62.06863883070810317, 48.89596633111685975, 20.11004999522056025 ) ) ;
#8845=CARTESIAN_POINT ( 'NONE',  ( -27.87283258141598097, 46.40806184526439893, 11.18159849702474240 ) ) ;
#8851=VERTEX_POINT ( 'NONE', #5173 ) ;
#8855=CARTESIAN_POINT ( 'NONE',  ( -13.44321664086546875, 61.83368541783048755, -1.838823801362371668 ) ) ;
#8857=CARTESIAN_POINT ( 'NONE',  ( 3.337188803346179178, 35.57729950087108506, -8.044583786737664610 ) ) ;
#8866=CARTESIAN_POINT ( 'NONE',  ( -67.17811141605125158, 49.99997012509656713, 0.3311688885648463310 ) ) ;
#8867=CARTESIAN_POINT ( 'NONE',  ( -17.88142570751413274, 67.52739394234649239, 16.89079266652326439 ) ) ;
#8870=CARTESIAN_POINT ( 'NONE',  ( -66.81138001472987753, 51.23444936853855580, 3.305681383735873613 ) ) ;
#8873=CARTESIAN_POINT ( 'NONE',  ( -41.16026710375170694, 50.89060761561553647, -20.69263693287480521 ) ) ;
#8876=CARTESIAN_POINT ( 'NONE',  ( 47.00000000000000000, 51.46446609406726935, 3.535533905932731091 ) ) ;
#8881=CARTESIAN_POINT ( 'NONE',  ( -43.75092013918801115, 59.45036911068460483, -5.422234973716651751 ) ) ;
#8890=CARTESIAN_POINT ( 'NONE',  ( 34.00000000000000000, 59.99999999999998579, 0.000000000000000000 ) ) ;
#8891=CARTESIAN_POINT ( 'NONE',  ( 25.24065896695082145, 55.02620812721863786, 0.001656341455649923368 ) ) ;
#8897=CARTESIAN_POINT ( 'NONE',  ( -61.59556246352555320, 52.94114603458827872, 20.93095456750423722 ) ) ;
#8899=CARTESIAN_POINT ( 'NONE',  ( -20.96936038908104649, 62.08580392802151948, 19.80242024469750817 ) ) ;
#8900=CARTESIAN_POINT ( 'NONE',  ( -54.03632049363248768, 68.19182434251506209, 4.719955684811743879 ) ) ;
#8904=CARTESIAN_POINT ( 'NONE',  ( 12.52240408941406535, 44.41801188983610871, 18.37272825892985040 ) ) ;
#8909=CARTESIAN_POINT ( 'NONE',  ( 8.759403238133714353, 55.01273213413052332, -0.01040348312344842492 ) ) ;
#8911=CARTESIAN_POINT ( 'NONE',  ( -9.506476073891887424, 72.54341816039358548, -11.73172419143293865 ) ) ;
#8921=CARTESIAN_POINT ( 'NONE',  ( -52.88146049032556562, 73.03766007303350705, 10.81102556547625149 ) ) ;
#8924=AXIS2_PLACEMENT_3D ( 'NONE', #7393, #3975, #5723 ) ;
#8925=CARTESIAN_POINT ( 'NONE',  ( -69.14775524013775510, 50.25531755529721778, 1.611686515444774148 ) ) ;
#8927=EDGE_CURVE ( 'NONE', #2139, #7152, #2431, .T. ) ;
#8929=DIRECTION ( 'NONE',  ( 0.000000000000000000, 0.000000000000000000, -1.000000000000000000 ) ) ;
#8930=CARTESIAN_POINT ( 'NONE',  ( -69.52691976458234535, 34.01892180236649921, 2.749684864678113794 ) ) ;
#8934=ORIENTED_EDGE ( 'NONE', *, *, #7678, .T. ) ;
#8939=CARTESIAN_POINT ( 'NONE',  ( -59.79192388697324390, 53.29971140327118206, 6.792174639222999133 ) ) ;
#8944=EDGE_CURVE ( 'NONE', #760, #8109, #11440, .T. ) ;
#8948=VERTEX_POINT ( 'NONE', #7156 ) ;
#8954=CARTESIAN_POINT ( 'NONE',  ( 37.00000000000000000, 55.00000000000000000, 0.000000000000000000 ) ) ;
#8960=CARTESIAN_POINT ( 'NONE',  ( -17.00978866326984473, 58.05348413988616585, 3.972925965357411826 ) ) ;
#8962=EDGE_LOOP ( 'NONE', ( #8753, #9794 ) ) ;
#8963=CARTESIAN_POINT ( 'NONE',  ( -21.83980934632623772, 59.12499887129341403, 20.69724524603370597 ) ) ;
#8966=ORIENTED_EDGE ( 'NONE', *, *, #5408, .T. ) ;
#8972=CARTESIAN_POINT ( 'NONE',  ( -58.75094087149691546, 58.30862544132050118, 6.191974367482877106 ) ) ;
#8974=CARTESIAN_POINT ( 'NONE',  ( -14.52231952541034943, 75.43188300159135906, 5.490993919093054565 ) ) ;
#8975=CARTESIAN_POINT ( 'NONE',  ( -3.477628190354089099, 49.49309465598528845, -20.46958112014059950 ) ) ;
#8981=CARTESIAN_POINT ( 'NONE',  ( -68.34104732181950226, 33.99448141944334623, 0.006743540747238889813 ) ) ;
#8983=CARTESIAN_POINT ( 'NONE',  ( -42.66281101964754896, 63.04450918361814615, -19.42252581123130639 ) ) ;
#8991=CARTESIAN_POINT ( 'NONE',  ( 6.288736434038950662, 50.50500022705934811, 2.214244300018950895 ) ) ;
#8999=CARTESIAN_POINT ( 'NONE',  ( -0.6792758137180379130, 53.69893887388462872, -4.838731147744609551 ) ) ;
#9000=CARTESIAN_POINT ( 'NONE',  ( 6.077181813707832170, 41.04144508200626262, -1.373101212108361002 ) ) ;
#9010=CARTESIAN_POINT ( 'NONE',  ( -51.87153091508479719, 55.00409571353115012, 0.001995793859737243683 ) ) ;
#9015=CARTESIAN_POINT ( 'NONE',  ( -10.59643185551853151, 59.93469145766130879, -0.8217785073578240951 ) ) ;
#9017=CARTESIAN_POINT ( 'NONE',  ( -55.73751408985167899, 71.24607175163586703, 13.33484869932101269 ) ) ;
#9019=CARTESIAN_POINT ( 'NONE',  ( -36.18906244468503530, 38.22373822049622305, -12.89330079981896482 ) ) ;
#9023=ORIENTED_EDGE ( 'NONE', *, *, #4409, .F. ) ;
#9025=CARTESIAN_POINT ( 'NONE',  ( 36.99999999999999289, 45.00000000000001421, 1.224646799147351679E-15 ) ) ;
#9030=CARTESIAN_POINT ( 'NONE',  ( -7.170201598857286029, 54.99827432856260145, 0.003516170034810423960 ) ) ;
#9032=CARTESIAN_POINT ( 'NONE',  ( -7.452025537132175970, 67.52141018531283123, -16.88433180000173195 ) ) ;
#9033=CARTESIAN_POINT ( 'NONE',  ( -42.03064326886630653, 53.96872019721284630, -20.99365203016559178 ) ) ;
#9034=CARTESIAN_POINT ( 'NONE',  ( -78.00000000000000000, 54.99999999999999289, 0.000000000000000000 ) ) ;
#9037=ORIENTED_EDGE ( 'NONE', *, *, #1824, .F. ) ;
#9043=CARTESIAN_POINT ( 'NONE',  ( -57.87010688772392086, 58.05147143109211072, 3.974243011944121662 ) ) ;
#9046=FACE_OUTER_BOUND ( 'NONE', #7789, .T. ) ;
#9054=CARTESIAN_POINT ( 'NONE',  ( 16.79375990066182922, 56.83099525978803257, 13.97545931189135793 ) ) ;
#9062=CARTESIAN_POINT ( 'NONE',  ( -36.87377965891732146, 50.66043048872463572, -2.505278942661100849 ) ) ;
#9065=CARTESIAN_POINT ( 'NONE',  ( -37.56959447096606652, 54.99363160768596259, -0.01863072254107098896 ) ) ;
#9067=CYLINDRICAL_SURFACE ( 'NONE', #4615, 9.999999999999987566 ) ;
#9068=CARTESIAN_POINT ( 'NONE',  ( -24.01777539311168397, 52.49472557160137143, 4.339384516595543140 ) ) ;
#9072=CARTESIAN_POINT ( 'NONE',  ( -62.73530513678402087, 48.89572068339310107, 20.11073150603193938 ) ) ;
#9074=CARTESIAN_POINT ( 'NONE',  ( 4.329456757236127551, 33.97246960341611555, -0.0004353087921988608999 ) ) ;
#9078=CARTESIAN_POINT ( 'NONE',  ( -28.67054321954914542, 35.57240153874681710, 8.046710727719679213 ) ) ;
#9082=CARTESIAN_POINT ( 'NONE',  ( -61.66652652224714615, 54.99971167242890147, 7.011010121665977479 ) ) ;
#9084=CARTESIAN_POINT ( 'NONE',  ( -4.274947514841225704, 57.05942961895281229, -21.01658053370092816 ) ) ;
#9086=CARTESIAN_POINT ( 'NONE',  ( 2.881307801134362023, 34.60859193927083055, -5.107160905361891601 ) ) ;
#9092=CARTESIAN_POINT ( 'NONE',  ( -37.90726342759032264, 55.01040348274680269, 0.01273213325553751787 ) ) ;
#9093=CARTESIAN_POINT ( 'NONE',  ( -36.26619597527190564, 52.35453385845364238, -4.245986690839498756 ) ) ;
#9109=CARTESIAN_POINT ( 'NONE',  ( -18.12197315986341550, 62.20417759841708261, 12.01780937852947595 ) ) ;
#9118=CARTESIAN_POINT ( 'NONE',  ( -23.75939059330988457, 54.98844314865997518, 0.02356513468685287119 ) ) ;
#9122=CARTESIAN_POINT ( 'NONE',  ( -8.462009850179832426, 59.33805624513391308, -2.507821275865560029 ) ) ;
#9128=CARTESIAN_POINT ( 'NONE',  ( -12.81092923270300865, 75.46953867936616689, -5.507006106411301616 ) ) ;
#9134=CARTESIAN_POINT ( 'NONE',  ( -32.17314280228392676, 34.29902663375150240, -4.109485608336678197 ) ) ;
#9139=CARTESIAN_POINT ( 'NONE',  ( -64.00030959431065014, 52.31932374249372941, 6.472111605756746933 ) ) ;
#9142=CARTESIAN_POINT ( 'NONE',  ( -40.69731036757077192, 53.96875818098316557, -20.99256918425749063 ) ) ;
#9143=CARTESIAN_POINT ( 'NONE',  ( 1.697306494461763959, 35.98764835359665426, -8.991780390316415961 ) ) ;
#9148=ORIENTED_EDGE ( 'NONE', *, *, #10688, .T. ) ;
#9150=CARTESIAN_POINT ( 'NONE',  ( -31.38106053236869286, 55.00524807308060105, -0.001787053225003424348 ) ) ;
#9151=CARTESIAN_POINT ( 'NONE',  ( -31.01894826520979365, 49.99999999999997868, -0.6617035227858814039 ) ) ;
#9163=DIRECTION ( 'NONE',  ( -6.033820786006286457E-17, 1.000000000000000000, 0.000000000000000000 ) ) ;
#9165=CARTESIAN_POINT ( 'NONE',  ( -6.128719672236011107, 58.04896597338179021, -3.976206575877460736 ) ) ;
#9166=VECTOR ( 'NONE', #11220, 1000.000000000000000 ) ;
#9167=CARTESIAN_POINT ( 'NONE',  ( -27.16357883943494400, 43.30581957307868635, 7.809306310971448895 ) ) ;
#9173=VECTOR ( 'NONE', #4882, 1000.000000000000000 ) ;
#9178=CARTESIAN_POINT ( 'NONE',  ( -55.09748469029145923, 54.99365593231603810, -0.01917390278371958537 ) ) ;
#9180=AXIS2_PLACEMENT_3D ( 'NONE', #7596, #391, #6821 ) ;
#9182=CARTESIAN_POINT ( 'NONE',  ( -23.62122360972324842, 52.78556759016737487, 4.494981739694955181 ) ) ;
#9183=ORIENTED_EDGE ( 'NONE', *, *, #2058, .F. ) ;
#9186=CARTESIAN_POINT ( 'NONE',  ( -8.785358865379802040, 67.52185545713140868, -16.88477868139494831 ) ) ;
#9190=CARTESIAN_POINT ( 'NONE',  ( -40.92935782463053584, 57.05919160630219977, -20.93299540428984429 ) ) ;
#9195=CARTESIAN_POINT ( 'NONE',  ( -8.872461119604453827, 57.50149492254836758, -4.332372781979526799 ) ) ;
#9196=CARTESIAN_POINT ( 'NONE',  ( 0.2748429140369315071, 38.70467982241823535, -13.38321124372595783 ) ) ;
#9198=CARTESIAN_POINT ( 'NONE',  ( -26.18898619208348677, 42.10803998828228600, 16.77528611580634887 ) ) ;
#9200=CARTESIAN_POINT ( 'NONE',  ( 2.595920079249742329, 34.88763922991881827, -6.102757042485290384 ) ) ;
#9204=CARTESIAN_POINT ( 'NONE',  ( -78.00000000000000000, 59.99999999999998579, 0.000000000000000000 ) ) ;
#9209=CARTESIAN_POINT ( 'NONE',  ( -30.50353493236575630, 55.00370654185008590, -0.001266073661171608069 ) ) ;
#9216=CARTESIAN_POINT ( 'NONE',  ( 11.81093755974026394, 42.10901286868706705, 16.77394813616862734 ) ) ;
#9219=CARTESIAN_POINT ( 'NONE',  ( 3.963041193916334137, 50.00000000000020606, 0.3308364528915549441 ) ) ;
#9223=PLANE ( 'NONE',  #5581 ) ;
#9226=CARTESIAN_POINT ( 'NONE',  ( 14.46039494637405909, 51.34337453854569588, 13.61230544799882480 ) ) ;
#9237=CARTESIAN_POINT ( 'NONE',  ( -29.12853506694033356, 55.00558571566143229, 0.0002252870501606599272 ) ) ;
#9246=CARTESIAN_POINT ( 'NONE',  ( 5.506399570602333426, 34.30736306936326230, 4.109392375493936100 ) ) ;
#9249=CARTESIAN_POINT ( 'NONE',  ( -1.477628194636992243, 49.49121550494065502, -20.47411891050684218 ) ) ;
#9250=CARTESIAN_POINT ( 'NONE',  ( -45.81092964171354964, 71.80742102382775727, -12.92463648794852205 ) ) ;
#9257=CARTESIAN_POINT ( 'NONE',  ( -37.85565285117030498, 44.43519602072407082, -18.33024205669471840 ) ) ;
#9258=CARTESIAN_POINT ( 'NONE',  ( -55.45210586135002728, 71.88485191958531573, 12.52183031059725771 ) ) ;
#9263=CARTESIAN_POINT ( 'NONE',  ( -34.28557208676265589, 54.99469277422922175, -0.0007481125482429651277 ) ) ;
#9264=CARTESIAN_POINT ( 'NONE',  ( -48.90475262238859244, 59.99999999999997158, -9.564595459368971197E-12 ) ) ;
#9267=CARTESIAN_POINT ( 'NONE',  ( -54.92282199211652483, 67.36828978179006810, 6.609266281412864430 ) ) ;
#9269=CARTESIAN_POINT ( 'NONE',  ( 0.8557374297261139962, 42.07536394375442512, -16.80742094040031631 ) ) ;
#9279=CARTESIAN_POINT ( 'NONE',  ( -60.99710787470219486, 49.63646281896018309, 12.94522044443767683 ) ) ;
#9290=CARTESIAN_POINT ( 'NONE',  ( 19.44332440029096887, 58.51573196296779855, 6.093031587449661224 ) ) ;
#9297=ORIENTED_EDGE ( 'NONE', *, *, #11161, .T. ) ;
#9301=CARTESIAN_POINT ( 'NONE',  ( 2.881307801134362023, 34.60859193927083055, -5.107160905361891601 ) ) ;
#9308=CARTESIAN_POINT ( 'NONE',  ( -46.52239103091250172, 73.32882989972571863, -10.56393531560676102 ) ) ;
#9311=CARTESIAN_POINT ( 'NONE',  ( -32.17314280228392676, 34.29902663375150240, -4.109485608336678197 ) ) ;
#9313=DIRECTION ( 'NONE',  ( 1.000000000000000000, 6.033820786006286457E-17, -0.000000000000000000 ) ) ;
#9314=DIRECTION ( 'NONE',  ( -1.000000000000000000, -9.813077866773612233E-16, 0.000000000000000000 ) ) ;
#9315=CARTESIAN_POINT ( 'NONE',  ( 2.881307801134362023, 34.60859193927083055, -5.107160905361891601 ) ) ;
#9317=CARTESIAN_POINT ( 'NONE',  ( -37.14429486108867451, 42.07659820469130096, -16.80634109873993864 ) ) ;
#9319=CARTESIAN_POINT ( 'NONE',  ( -44.66281104389123868, 63.04473320575852568, -19.42304942373100829 ) ) ;
#9326=CARTESIAN_POINT ( 'NONE',  ( -43.90973736884477319, 55.00080601838077143, -0.005934653685857244065 ) ) ;
#9327=CARTESIAN_POINT ( 'NONE',  ( -40.35278372931369262, 55.66209291482490329, -4.999970240424343793 ) ) ;
#9330=CARTESIAN_POINT ( 'NONE',  ( -9.750467871106947015, 59.44169190721913765, -5.412448594069168450 ) ) ;
#9332=CARTESIAN_POINT ( 'NONE',  ( -2.188986190505546769, 52.25407376895000056, -20.97627476078892528 ) ) ;
#9333=UNCERTAINTY_MEASURE_WITH_UNIT (LENGTH_MEASURE( 1.000000000000000082E-05 ), #2744, 'distance_accuracy_value', 'NONE');
#9344=CARTESIAN_POINT ( 'NONE',  ( 21.14436220910852882, 71.77416011014268804, 12.89076390558360075 ) ) ;
#9353=DIRECTION ( 'NONE',  ( -6.033820786006286457E-17, 1.000000000000000000, 0.000000000000000000 ) ) ;
#9355=CARTESIAN_POINT ( 'NONE',  ( 15.55675285225959570, 54.08367678788073363, 7.025375982562417576 ) ) ;
#9360=DIRECTION ( 'NONE',  ( -1.000000000000000000, -0.000000000000000000, -0.000000000000000000 ) ) ;
#9363=CARTESIAN_POINT ( 'NONE',  ( -61.00490302436042356, 55.00059028654953153, 21.02810969917934614 ) ) ;
#9366=CARTESIAN_POINT ( 'NONE',  ( -61.32723930490969622, 46.95308112547827051, 19.41976192622660946 ) ) ;
#9374=CARTESIAN_POINT ( 'NONE',  ( 22.99999999999999645, 76.00000000000000000, 0.000000000000000000 ) ) ;
#9376=CARTESIAN_POINT ( 'NONE',  ( -50.94162072875351299, 76.01658590998553677, 2.059423418002142459 ) ) ;
#9377=CARTESIAN_POINT ( 'NONE',  ( -65.06671514604981610, 41.61929618219224380, 16.30332023460171698 ) ) ;
#9379=AXIS2_PLACEMENT_3D ( 'NONE', #8494, #3936, #6588 ) ;
#9388=CARTESIAN_POINT ( 'NONE',  ( 53.00000000000000000, 51.46446609406726935, 3.535533905932731091 ) ) ;
#9392=CARTESIAN_POINT ( 'NONE',  ( -64.83840380677510495, 47.18714368648432611, 11.70375861309407206 ) ) ;
#9394=CARTESIAN_POINT ( 'NONE',  ( 0.1442708919848544047, 44.43605983923426805, -18.32883121229183487 ) ) ;
#9403=VERTEX_POINT ( 'NONE', #3179 ) ;
#9405=CARTESIAN_POINT ( 'NONE',  ( -41.74394153288059783, 59.06666331196394282, -13.40395870027933078 ) ) ;
#9407=ADVANCED_FACE ( 'NONE', ( #9644 ), #5047, .T. ) ;
#9414=CARTESIAN_POINT ( 'NONE',  ( -39.98517722295121501, 52.49184747003998552, -4.337707995793770976 ) ) ;
#9417=CARTESIAN_POINT ( 'NONE',  ( 8.750843404857064911, 48.25223522016324296, 2.051079653697085892 ) ) ;
#9419=CYLINDRICAL_SURFACE ( 'NONE', #1073, 2.999999999999999112 ) ;
#9425=CARTESIAN_POINT ( 'NONE',  ( -29.49360042904642043, 37.45509264529403737, 11.71531283165970727 ) ) ;
#9428=CARTESIAN_POINT ( 'NONE',  ( -52.88146049032556562, 73.03766007303350705, 10.81102556547625149 ) ) ;
#9434=CARTESIAN_POINT ( 'NONE',  ( -1.871122143093896906, 51.94779910732768258, -3.973801861892843235 ) ) ;
#9437=CARTESIAN_POINT ( 'NONE',  ( 15.85562909902672679, 60.50729566700048423, 20.47119405379366697 ) ) ;
#9438=CARTESIAN_POINT ( 'NONE',  ( 11.79372827400108470, 51.34087032111902715, 13.61835106791356154 ) ) ;
#9441=CARTESIAN_POINT ( 'NONE',  ( -15.09523335307150838, 60.00000000000000000, 4.640896189903090912E-12 ) ) ;
#9444=ORIENTED_EDGE ( 'NONE', *, *, #48, .T. ) ;
#9452=CARTESIAN_POINT ( 'NONE',  ( -63.96363525012968410, 49.00358019864930981, 12.67571071499552282 ) ) ;
#9453=ORIENTED_EDGE ( 'NONE', *, *, #18, .T. ) ;
#9455=CARTESIAN_POINT ( 'NONE',  ( -41.21475901749523274, 58.08538884819615333, -20.80179922188357011 ) ) ;
#9461=EDGE_CURVE ( 'NONE', #2759, #7749, #4793, .T. ) ;
#9467=CARTESIAN_POINT ( 'NONE',  ( -59.54425338440577775, 52.94308673282063182, 13.86869692379441510 ) ) ;
#9475=CARTESIAN_POINT ( 'NONE',  ( -47.37975114575861824, 58.30660270781542920, -3.764775390512491438 ) ) ;
#9477=CARTESIAN_POINT ( 'NONE',  ( -20.41758684020055981, 55.68721290480836217, 6.980984518528451588 ) ) ;
#9485=CARTESIAN_POINT ( 'NONE',  ( -40.60828084101493829, 48.86090744392433294, -20.20262880343927847 ) ) ;
#9489=CARTESIAN_POINT ( 'NONE',  ( -70.34104699118840642, 33.99562393659799397, 0.006612473344882377653 ) ) ;
#9496=CARTESIAN_POINT ( 'NONE',  ( -44.07074648197151845, 61.10275710191199749, -20.11236068975357938 ) ) ;
#9498=CARTESIAN_POINT ( 'NONE',  ( 4.403976020759948540, 34.06825102507477965, -2.059153462500010967 ) ) ;
#9499=CARTESIAN_POINT ( 'NONE',  ( 2.544693516836439073, 41.40683613508774386, -3.404232400632562161 ) ) ;
#9501=LINE ( 'NONE', #8548, #6239 ) ;
#9509=VECTOR ( 'NONE', #5604, 1000.000000000000000 ) ;
#9511=CARTESIAN_POINT ( 'NONE',  ( -28.22334563455873635, 50.71039758802199771, 5.585597018820382509 ) ) ;
#9513=ORIENTED_EDGE ( 'NONE', *, *, #10019, .T. ) ;
#9514=CARTESIAN_POINT ( 'NONE',  ( -53.45210586504737904, 71.88419113761085555, 12.52116934359859002 ) ) ;
#9527=CARTESIAN_POINT ( 'NONE',  ( 4.881307793505825110, 34.60946683332392126, -5.106800360247272685 ) ) ;
#9536=CARTESIAN_POINT ( 'NONE',  ( -45.81573735730770380, 57.21589932804895540, -4.494086191879637759 ) ) ;
#9539=EDGE_CURVE ( 'NONE', #7152, #11420, #3193, .T. ) ;
#9540=CARTESIAN_POINT ( 'NONE',  ( 5.541412553157611498, 48.20653848766852434, -1.700702987377777253 ) ) ;
#9548=CARTESIAN_POINT ( 'NONE',  ( -52.27495405780593529, 76.01412898031726684, 2.059423305703688811 ) ) ;
#9555=ORIENTED_EDGE ( 'NONE', *, *, #11787, .F. ) ;
#9558=CARTESIAN_POINT ( 'NONE',  ( -34.17314261869798742, 34.29999169977881479, -4.109493429249395646 ) ) ;
#9560=CARTESIAN_POINT ( 'NONE',  ( -0.4775959007562765590, 42.07767894935109609, -16.80510553145697727 ) ) ;
#9562=CARTESIAN_POINT ( 'NONE',  ( -13.87290721739879551, 68.98200347986859526, -1.830994221428368540 ) ) ;
#9564=FACE_OUTER_BOUND ( 'NONE', #3858, .T. ) ;
#9569=LINE ( 'NONE', #8675, #7017 ) ;
#9570=DIRECTION ( 'NONE',  ( 0.000000000000000000, -1.000000000000000000, 0.000000000000000000 ) ) ;
#9572=CARTESIAN_POINT ( 'NONE',  ( -20.24961059810222963, 59.45058868119262740, 5.422033872742003879 ) ) ;
#9574=CARTESIAN_POINT ( 'NONE',  ( -29.26269115883859939, 34.87241548204915631, 6.108265559058850158 ) ) ;
#9580=DIRECTION ( 'NONE',  ( 1.000000000000000000, 6.033820786006286457E-17, -0.000000000000000000 ) ) ;
#9586=CARTESIAN_POINT ( 'NONE',  ( -26.94161418247137263, 38.68192823000178038, 13.40559829713685502 ) ) ;
#9590=LINE ( 'NONE', #5952, #7624 ) ;
#9598=ORIENTED_EDGE ( 'NONE', *, *, #349, .T. ) ;
#9601=CARTESIAN_POINT ( 'NONE',  ( -27.70870029355219089, 48.67231285529162932, 2.993251960717111082 ) ) ;
#9606=ORIENTED_EDGE ( 'NONE', *, *, #3224, .F. ) ;
#9612=CARTESIAN_POINT ( 'NONE',  ( 1.907306313148354304, 54.98265195905499780, -0.01969434134204536141 ) ) ;
#9617=CARTESIAN_POINT ( 'NONE',  ( -44.66281104389123868, 63.04473320575852568, -19.42304942373100829 ) ) ;
#9619=CARTESIAN_POINT ( 'NONE',  ( -12.14426256746178368, 75.47105121598427502, -5.507632465234872043 ) ) ;
#9620=CARTESIAN_POINT ( 'NONE',  ( -20.78863981635950609, 62.20466253127742817, 12.01897416180004896 ) ) ;
#9629=CARTESIAN_POINT ( 'NONE',  ( -47.08425347821636819, 59.45470633346049993, -5.426572237033094659 ) ) ;
#9631=CARTESIAN_POINT ( 'NONE',  ( -17.00387655282055377, 69.86881140706658755, 14.86941770366936311 ) ) ;
#9632=CARTESIAN_POINT ( 'NONE',  ( 15.18896243380506306, 60.50666922109576262, 20.46968130491651650 ) ) ;
#9641=CARTESIAN_POINT ( 'NONE',  ( 0.8557374297261139962, 42.07536394375442512, -16.80742094040031631 ) ) ;
#9642=CYLINDRICAL_SURFACE ( 'NONE', #1170, 4.999999999999984013 ) ;
#9644=FACE_OUTER_BOUND ( 'NONE', #5304, .T. ) ;
#9654=CARTESIAN_POINT ( 'NONE',  ( -35.77658090492886345, 50.68024773144422568, -5.615629700006128822 ) ) ;
#9656=DIRECTION ( 'NONE',  ( 0.000000000000000000, 1.000000000000000000, 0.000000000000000000 ) ) ;
#9657=ORIENTED_EDGE ( 'NONE', *, *, #3310, .F. ) ;
#9665=PLANE ( 'NONE',  #6747 ) ;
#9666=CARTESIAN_POINT ( 'NONE',  ( -16.57640557450304897, 55.00618966384792685, 0.007491359115028465437 ) ) ;
#9672=CARTESIAN_POINT ( 'NONE',  ( -42.92935705524211443, 57.05913440163546113, -20.93112575922673102 ) ) ;
#9675=CARTESIAN_POINT ( 'NONE',  ( -7.262690645865875538, 64.91264328142536044, -18.55041054278238022 ) ) ;
#9676=CARTESIAN_POINT ( 'NONE',  ( -0.07137196575059991110, 44.13905398550945591, -8.918958607883686440 ) ) ;
#9680=CARTESIAN_POINT ( 'NONE',  ( -23.64880231868481175, 55.66116299125641831, 5.000007605738006511 ) ) ;
#9683=CARTESIAN_POINT ( 'NONE',  ( 21.85574933723554736, 73.37275400661043534, 10.58193396047185075 ) ) ;
#9686=CARTESIAN_POINT ( 'NONE',  ( -27.44324756452158098, 51.46806551970854571, 6.132376716174161579 ) ) ;
#9688=CARTESIAN_POINT ( 'NONE',  ( -40.92935782463053584, 57.05919160630219977, -20.93299540428984429 ) ) ;
#9695=ORIENTED_EDGE ( 'NONE', *, *, #18, .F. ) ;
#9699=CARTESIAN_POINT ( 'NONE',  ( -28.67054321954914542, 35.57240153874681710, 8.046710727719679213 ) ) ;
#9707=CARTESIAN_POINT ( 'NONE',  ( -67.56971494453328830, 50.00000002031717372, -0.0004507456344833478141 ) ) ;
#9712=CARTESIAN_POINT ( 'NONE',  ( -66.11067862173452170, 48.15427919969674520, 1.842099731909419225 ) ) ;
#9721=CARTESIAN_POINT ( 'NONE',  ( -6.090330045190794905, 54.99253937026119843, 0.007033857285447905894 ) ) ;
#9726=CARTESIAN_POINT ( 'NONE',  ( -54.00383531698385298, 74.42670172875287449, 8.047314657126378279 ) ) ;
#9727=EDGE_LOOP ( 'NONE', ( #4939, #5263, #434 ) ) ;
#9728=CARTESIAN_POINT ( 'NONE',  ( -45.72515810441178274, 68.38234357726757651, -16.29445369018955247 ) ) ;
#9729=CARTESIAN_POINT ( 'NONE',  ( 1.369680300758778113, 42.32355992005446410, -5.995427644676592394 ) ) ;
#9735=CARTESIAN_POINT ( 'NONE',  ( 7.506399388638331338, 34.30832474160909129, 4.109400874309620200 ) ) ;
#9736=EDGE_CURVE ( 'NONE', #1195, #4551, #11408, .T. ) ;
#9739=CARTESIAN_POINT ( 'NONE',  ( 20.70698219299188381, 58.30206649714182277, 3.768798166023678231 ) ) ;
#9740=CARTESIAN_POINT ( 'NONE',  ( -56.41713135980065630, 60.41248846187414756, 4.441724532788772883 ) ) ;
#9741=CONICAL_SURFACE ( 'NONE', #4395, 2.999999999999995559, 0.7853981633974420618 ) ;
#9743=CARTESIAN_POINT ( 'NONE',  ( 5.969356325850132983, 34.00743083263078859, 1.031241799122481595 ) ) ;
#9754=CARTESIAN_POINT ( 'NONE',  ( 2.826857198123298165, 37.44742646213195769, -11.71858918393001225 ) ) ;
#9760=CARTESIAN_POINT ( 'NONE',  ( -24.47759590008010377, 52.25445690686086664, 21.01882782503509262 ) ) ;
#9767=VERTEX_POINT ( 'NONE', #10402 ) ;
#9769=CARTESIAN_POINT ( 'NONE',  ( -60.08385138347627219, 52.96922280571201469, 6.695818664272940701 ) ) ;
#9772=CARTESIAN_POINT ( 'NONE',  ( -14.70500487297517189, 60.00000000000030553, -0.3308759158401262668 ) ) ;
#9781=CARTESIAN_POINT ( 'NONE',  ( 4.997868933204849817, 55.00264723353835450, 0.001346135474403307910 ) ) ;
#9789=CARTESIAN_POINT ( 'NONE',  ( -59.27472368810988002, 61.13901599248961105, 20.20251803659174783 ) ) ;
#9791=CARTESIAN_POINT ( 'NONE',  ( -32.32947787139347895, 33.97704578748628990, 0.0005171865318368603498 ) ) ;
#9792=CARTESIAN_POINT ( 'NONE',  ( -20.21146696499166140, 63.35170862394775071, 11.26075774480146485 ) ) ;
#9794=ORIENTED_EDGE ( 'NONE', *, *, #10688, .F. ) ;
#9796=CARTESIAN_POINT ( 'NONE',  ( 8.058385817489730485, 34.79396711235183659, 6.140502173211014103 ) ) ;
#9799=CARTESIAN_POINT ( 'NONE',  ( 23.03641490397931335, 59.49166983161503452, 2.221310855399595496 ) ) ;
#9800=CARTESIAN_POINT ( 'NONE',  ( -65.75072559461156629, 50.54239926659131044, 5.429416014682115765 ) ) ;
#9802=CARTESIAN_POINT ( 'NONE',  ( 5.662790106042886684, 33.97208755798592961, -0.0004309138471297446066 ) ) ;
#9814=CARTESIAN_POINT ( 'NONE',  ( -52.59603425219209782, 73.55155261293346314, 9.913157997185967574 ) ) ;
#9823=CARTESIAN_POINT ( 'NONE',  ( 19.51996453321225644, 59.49466458524579338, 2.214906497190253010 ) ) ;
#9828=EDGE_CURVE ( 'NONE', #1911, #3047, #3277, .T. ) ;
#9831=CARTESIAN_POINT ( 'NONE',  ( -45.10988329347496517, 60.61560339207529324, -4.319777640813139641 ) ) ;
#9841=CARTESIAN_POINT ( 'NONE',  ( -6.668797733382348270, 54.99774328067935159, 0.001930581088264634107 ) ) ;
#9847=CARTESIAN_POINT ( 'NONE',  ( -44.30269363598408461, 63.99200565043310007, -19.01284557474750514 ) ) ;
#9856=CARTESIAN_POINT ( 'NONE',  ( 14.87104979758787771, 53.70723891340239220, 4.840877117755912451 ) ) ;
#9857=CARTESIAN_POINT ( 'NONE',  ( -8.047727199116865293, 54.99755268931162533, 0.004974585571924257203 ) ) ;
#9859=CARTESIAN_POINT ( 'NONE',  ( -12.18906244258289995, 75.97791289299129858, -2.745668048143513396 ) ) ;
#9860=CARTESIAN_POINT ( 'NONE',  ( -30.36397657560652874, 35.99904827701746513, 8.986701095552454888 ) ) ;
#9869=CARTESIAN_POINT ( 'NONE',  ( -61.32723930490969622, 46.95308112547827051, 19.41976192622660946 ) ) ;
#9875=CARTESIAN_POINT ( 'NONE',  ( 7.851389403161795677, 51.23265128290481840, 3.303652424085503636 ) ) ;
#9877=LINE ( 'NONE', #1673, #2679 ) ;
#9882=CARTESIAN_POINT ( 'NONE',  ( 7.095683716263478047, 50.00000000000005684, 2.757939276259992832E-15 ) ) ;
#9884=CARTESIAN_POINT ( 'NONE',  ( -5.001868413209209940, 60.36545409722314304, -12.95245650687548356 ) ) ;
#9899=CARTESIAN_POINT ( 'NONE',  ( -29.42366337843931490, 55.01024914994471260, 0.0003017736481339514825 ) ) ;
#9903=ORIENTED_EDGE ( 'NONE', *, *, #6156, .F. ) ;
#9904=CARTESIAN_POINT ( 'NONE',  ( -15.46272266344517909, 58.97603181275015771, 3.049243307324925656 ) ) ;
#9907=CARTESIAN_POINT ( 'NONE',  ( -53.92936707256667717, 73.55041509984243930, 9.912644826577484025 ) ) ;
#9909=AXIS2_PLACEMENT_3D ( 'NONE', #10647, #4987, #1500 ) ;
#9912=CARTESIAN_POINT ( 'NONE',  ( 25.76190476190475565, 59.99999999999995026, 0.000000000000000000 ) ) ;
#9916=CARTESIAN_POINT ( 'NONE',  ( -0.1631717787953173293, 54.99775794017483577, -0.001150061841714329494 ) ) ;
#9918=CARTESIAN_POINT ( 'NONE',  ( -58.69833756168564065, 56.03204939003842355, 20.99267139547387373 ) ) ;
#9919=CARTESIAN_POINT ( 'NONE',  ( -30.67054324275970600, 35.57292846186890500, 8.046485333435041909 ) ) ;
#9921=VECTOR ( 'NONE', #3885, 1000.000000000000000 ) ;
#9930=DIRECTION ( 'NONE',  ( 1.000000000000000000, 6.033820786006286457E-17, -0.000000000000000000 ) ) ;
#9933=CARTESIAN_POINT ( 'NONE',  ( -53.21169738097692203, 59.96713617643348471, 0.6587253374105324077 ) ) ;
#9935=CARTESIAN_POINT ( 'NONE',  ( 36.99999999999999289, 45.00000000000001421, 1.224646799147351679E-15 ) ) ;
#9945=CARTESIAN_POINT ( 'NONE',  ( -1.127104549820378221, 51.32464662373498498, -13.65769093838479442 ) ) ;
#9953=EDGE_CURVE ( 'NONE', #4670, #3266, #6662, .T. ) ;
#9956=CARTESIAN_POINT ( 'NONE',  ( -49.23625742515549319, 55.01965444600840272, 0.001248010823296030226 ) ) ;
#9957=DIRECTION ( 'NONE',  ( 1.000000000000000000, 6.033820786006286457E-17, -0.000000000000000000 ) ) ;
#9960=CARTESIAN_POINT ( 'NONE',  ( -9.624147497243844995, 59.74499220970398028, -1.610198918108491029 ) ) ;
#9961=CARTESIAN_POINT ( 'NONE',  ( -62.45014759628331547, 49.89181376149021219, 20.39015500988638507 ) ) ;
#9963=CARTESIAN_POINT ( 'NONE',  ( -31.73741350946478335, 34.08379956678489009, 2.058435976334235473 ) ) ;
#9966=CIRCLE ( 'NONE', #6557, 4.999999999999997335 ) ;
#9970=CARTESIAN_POINT ( 'NONE',  ( -28.36397722366938012, 36.00052710555507218, 8.986026874162561739 ) ) ;
#9974=CARTESIAN_POINT ( 'NONE',  ( -8.331185513520907193, 55.00093008094477653, -0.001764911158480240083 ) ) ;
#9976=CARTESIAN_POINT ( 'NONE',  ( 0.1890707644848960145, 42.07652144655710913, -16.80626323592864324 ) ) ;
#9977=CARTESIAN_POINT ( 'NONE',  ( -29.49360042904642043, 37.45509264529403737, 11.71531283165970727 ) ) ;
#9981=ORIENTED_EDGE ( 'NONE', *, *, #5718, .F. ) ;
#9982=DIRECTION ( 'NONE',  ( 1.000000000000000000, 6.033820786006286457E-17, -0.000000000000000000 ) ) ;
#9983=CARTESIAN_POINT ( 'NONE',  ( -45.09032857029786356, 54.99712218131477925, 0.005861851983533778246 ) ) ;
#9984=CARTESIAN_POINT ( 'NONE',  ( -31.79252387391919754, 50.12764572993967249, -1.301498629944670249 ) ) ;
#9987=CARTESIAN_POINT ( 'NONE',  ( 36.99999999999999289, 55.00000000000000000, 0.000000000000000000 ) ) ;
#9988=CARTESIAN_POINT ( 'NONE',  ( -63.70414766735607515, 53.39330387528737987, 4.746099453471545715 ) ) ;
#9991=CARTESIAN_POINT ( 'NONE',  ( -31.04449509981424526, 50.50450958133799872, 2.213278473101321087 ) ) ;
#9992=CARTESIAN_POINT ( 'NONE',  ( -68.81799204399976588, 34.52608862562686909, 5.501299279293338174 ) ) ;
#9997=ORIENTED_EDGE ( 'NONE', *, *, #7600, .F. ) ;
#9998=CARTESIAN_POINT ( 'NONE',  ( -1.262803747101160834, 54.17797665385903372, -4.934652714417677721 ) ) ;
#9999=CARTESIAN_POINT ( 'NONE',  ( 0.4604261215510325744, 47.96020507958075285, -12.21094979895113219 ) ) ;
#10002=EDGE_CURVE ( 'NONE', #1948, #1442, #6685, .T. ) ;
#10009=CARTESIAN_POINT ( 'NONE',  ( -41.66879782724831927, 54.99865377049987103, 0.002647339441117046391 ) ) ;
#10011=CARTESIAN_POINT ( 'NONE',  ( -11.18084273084829583, 59.99169012976696536, -0.3319299593735249854 ) ) ;
#10012=ORIENTED_EDGE ( 'NONE', *, *, #3400, .T. ) ;
#10015=ORIENTED_EDGE ( 'NONE', *, *, #7600, .T. ) ;
#10016=CARTESIAN_POINT ( 'NONE',  ( -8.214759031591983174, 65.81066618478850216, -18.03675305545087681 ) ) ;
#10019=EDGE_CURVE ( 'NONE', #9403, #7593, #5702, .T. ) ;
#10022=CARTESIAN_POINT ( 'NONE',  ( -30.99614452189004155, 33.97742542711323921, 0.0005215828242728561687 ) ) ;
#10023=( NAMED_UNIT ( * ) SI_UNIT ( $, .STERADIAN. ) SOLID_ANGLE_UNIT ( ) );
#10028=CARTESIAN_POINT ( 'NONE',  ( -12.43046839200774656, 54.98819421727549184, 0.003555045980302951828 ) ) ;
#10030=CARTESIAN_POINT ( 'NONE',  ( -29.03064367431483817, 36.00003416271029266, 8.986251614625855311 ) ) ;
#10031=CARTESIAN_POINT ( 'NONE',  ( -32.40407992077046373, 34.08317752212569474, 2.058454929014103651 ) ) ;
#10038=PLANE ( 'NONE',  #11095 ) ;
#10039=CARTESIAN_POINT ( 'NONE',  ( -55.87153088905797915, 55.00233510441087503, 0.001258675581659554621 ) ) ;
#10040=CARTESIAN_POINT ( 'NONE',  ( -37.62597467746413571, 53.39124767624571888, -4.745502624100200073 ) ) ;
#10053=CARTESIAN_POINT ( 'NONE',  ( 52.99999999999999289, 55.00000000000000000, 2.999999999999999112 ) ) ;
#10054=CARTESIAN_POINT ( 'NONE',  ( -16.36967209184480865, 65.37984753263212667, 9.407486617481991331 ) ) ;
#10065=CARTESIAN_POINT ( 'NONE',  ( -54.49661136968474295, 55.00298157538451704, 0.003101384249735006544 ) ) ;
#10073=CARTESIAN_POINT ( 'NONE',  ( -68.15132479584509895, 34.52429035776697930, 5.502002828716508809 ) ) ;
#10079=CARTESIAN_POINT ( 'NONE',  ( -9.391823749396904120, 73.59702374900430755, -9.931971109272440756 ) ) ;
#10080=SURFACE_STYLE_USAGE ( .BOTH. , #3869 ) ;
#10081=CARTESIAN_POINT ( 'NONE',  ( -68.34104732181945963, 33.99448141944315438, 0.006743540747239065887 ) ) ;
#10083=CARTESIAN_POINT ( 'NONE',  ( -5.371237946277282127, 54.66875656801337158, -4.999992488715903960 ) ) ;
#10084=DIRECTION ( 'NONE',  ( 0.000000000000000000, 0.000000000000000000, 1.000000000000000000 ) ) ;
#10087=CARTESIAN_POINT ( 'NONE',  ( -42.73741365937004844, 61.10231602703586873, -20.11119678530976884 ) ) ;
#10088=CARTESIAN_POINT ( 'NONE',  ( -19.00387657603030078, 69.86840152515847535, 14.86901714484747750 ) ) ;
#10090=CARTESIAN_POINT ( 'NONE',  ( -30.23830917210572267, 50.00000000000000711, 1.120793995806890209E-14 ) ) ;
#10093=ADVANCED_FACE ( 'NONE', ( #6749 ), #5841, .T. ) ;
#10096=CARTESIAN_POINT ( 'NONE',  ( -37.09269367797786998, 54.98551036657900681, -0.007796657494142412992 ) ) ;
#10097=CARTESIAN_POINT ( 'NONE',  ( -30.23830917210572267, 50.00000000000000711, 1.120793995806890209E-14 ) ) ;
#10098=FACE_OUTER_BOUND ( 'NONE', #1939, .T. ) ;
#10102=ORIENTED_EDGE ( 'NONE', *, *, #6255, .F. ) ;
#10103=CARTESIAN_POINT ( 'NONE',  ( 4.881307793505825110, 34.60946683332392126, -5.106800360247272685 ) ) ;
#10114=EDGE_CURVE ( 'NONE', #3861, #3881, #514, .T. ) ;
#10115=CARTESIAN_POINT ( 'NONE',  ( -17.54480031048505495, 63.35260169467658642, 11.26165491496548832 ) ) ;
#10119=AXIS2_PLACEMENT_3D ( 'NONE', #7149, #3356, #2584 ) ;
#10124=CARTESIAN_POINT ( 'NONE',  ( -60.33684501428881930, 55.00322620591916944, -0.003862519133706141233 ) ) ;
#10130=CARTESIAN_POINT ( 'NONE',  ( 11.37836091825973561, 51.23382177081494149, 3.305048827278960211 ) ) ;
#10131=DIRECTION ( 'NONE',  ( 1.000000000000000000, 6.033820786006286457E-17, -0.000000000000000000 ) ) ;
#10133=CARTESIAN_POINT ( 'NONE',  ( -1.855729112296511385, 44.43418165317581980, -18.33336562707187412 ) ) ;
#10136=ORIENTED_EDGE ( 'NONE', *, *, #5408, .F. ) ;
#10137=DIRECTION ( 'NONE',  ( 1.000000000000000000, 6.033820786006286457E-17, 0.000000000000000000 ) ) ;
#10138=CARTESIAN_POINT ( 'NONE',  ( 4.003855478097921861, 35.57747403031575573, -8.044509115018048107 ) ) ;
#10140=( NAMED_UNIT ( * ) PLANE_ANGLE_UNIT ( ) SI_UNIT ( $, .RADIAN. ) );
#10141=CARTESIAN_POINT ( 'NONE',  ( -40.33720992201957500, 55.00042869323097960, -21.02810349118288258 ) ) ;
#10148=CARTESIAN_POINT ( 'NONE',  ( -17.36397700743563632, 70.57318608196271725, 14.11478994354440530 ) ) ;
#10151=CARTESIAN_POINT ( 'NONE',  ( -55.73751408985167899, 71.24607175163586703, 13.33484869932101269 ) ) ;
#10153=( NAMED_UNIT ( * ) SI_UNIT ( $, .STERADIAN. ) SOLID_ANGLE_UNIT ( ) );
#10159=LINE ( 'NONE', #11723, #3476 ) ;
#10160=CARTESIAN_POINT ( 'NONE',  ( -26.24059676141881781, 55.00778171745486134, -0.01448394145446873539 ) ) ;
#10166=CARTESIAN_POINT ( 'NONE',  ( -56.96367441743876725, 64.41719779848563121, 10.39011149079907526 ) ) ;
#10168=CARTESIAN_POINT ( 'NONE',  ( 2.826857198123298165, 37.44742646213195769, -11.71858918393001225 ) ) ;
#10178=DIRECTION ( 'NONE',  ( 1.000000000000000000, 6.033820786006286457E-17, -0.000000000000000000 ) ) ;
#10181=CARTESIAN_POINT ( 'NONE',  ( -55.73773073934312805, 61.61875917375134293, 12.39151048960789048 ) ) ;
#10185=EDGE_CURVE ( 'NONE', #9767, #1442, #7331, .T. ) ;
#10193=CARTESIAN_POINT ( 'NONE',  ( -0.7765809050102786548, 53.15807774253367057, -6.841262966262681822 ) ) ;
#10196=VERTEX_POINT ( 'NONE', #6315 ) ;
#10198=CYLINDRICAL_SURFACE ( 'NONE', #5180, 4.999999999999984013 ) ;
#10200=CARTESIAN_POINT ( 'NONE',  ( 9.810937555461070048, 42.10554236623130464, 16.77741859935663626 ) ) ;
#10204=CARTESIAN_POINT ( 'NONE',  ( -15.82693394478133797, 72.53700911420227726, 11.72543866452437733 ) ) ;
#10205=FILL_AREA_STYLE ('',( #2909 ) ) ;
#10206=DIRECTION ( 'NONE',  ( 1.000000000000000000, 6.033820786006286457E-17, 0.000000000000000000 ) ) ;
#10209=CARTESIAN_POINT ( 'NONE',  ( -4.208370785906845768, 53.70404148446576897, -4.840060944352733152 ) ) ;
#10212=CARTESIAN_POINT ( 'NONE',  ( -28.16026721702189306, 37.45568712642866416, 11.71507272220211071 ) ) ;
#10213=CARTESIAN_POINT ( 'NONE',  ( 21.87131398367523616, 69.01805473306414740, 1.834616117294233240 ) ) ;
#10221=CARTESIAN_POINT ( 'NONE',  ( -33.42366184627161374, 55.00651688198467326, 0.0004154897275390965193 ) ) ;
#10222=CARTESIAN_POINT ( 'NONE',  ( -49.29517856930504394, 60.00000000000064659, 0.3319123253646104055 ) ) ;
#10225=CARTESIAN_POINT ( 'NONE',  ( 4.833109902090660270, 48.10506029203823175, 1.369963280143046136 ) ) ;
#10237=CARTESIAN_POINT ( 'NONE',  ( 21.85574933723554736, 73.37275400661043534, 10.58193396047185075 ) ) ;
#10248=CARTESIAN_POINT ( 'NONE',  ( -16.33319360682722632, 59.95766673739793617, 4.958029769595817982 ) ) ;
#10258=CARTESIAN_POINT ( 'NONE',  ( -15.85565286160008469, 75.43490621471428881, 5.492246195135631837 ) ) ;
#10261=CARTESIAN_POINT ( 'NONE',  ( -55.50627899214600092, 66.73177265193905328, 17.54361557889675893 ) ) ;
#10271=CARTESIAN_POINT ( 'NONE',  ( -30.21475903739694857, 34.60120891540925925, 5.109855906315051044 ) ) ;
#10272=CARTESIAN_POINT ( 'NONE',  ( -54.00383531698385298, 74.42670172875287449, 8.047314657126378279 ) ) ;
#10275=VECTOR ( 'NONE', #1851, 1000.000000000000000 ) ;
#10276=CARTESIAN_POINT ( 'NONE',  ( -16.65533121350868839, 59.83994479200593020, 1.296523861810935374 ) ) ;
#10287=CARTESIAN_POINT ( 'NONE',  ( -56.66487171987550653, 64.91036822740932166, 9.909685932910122119 ) ) ;
#10289=CARTESIAN_POINT ( 'NONE',  ( 10.18903847268274276, 38.19250115101311849, 12.92455934260550521 ) ) ;
#10295=ORIENTED_EDGE ( 'NONE', *, *, #2800, .F. ) ;
#10299=CARTESIAN_POINT ( 'NONE',  ( -33.79373960940952770, 42.74365976533915301, -7.058510872263445535 ) ) ;
#10310=CARTESIAN_POINT ( 'NONE',  ( 20.22335381278353594, 59.31970004319295953, 5.615686161229384687 ) ) ;
#10316=CARTESIAN_POINT ( 'NONE',  ( 36.99999999999999289, 59.99999999999998579, 0.000000000000000000 ) ) ;
#10319=CARTESIAN_POINT ( 'NONE',  ( -44.66281104389123868, 63.04473320575852568, -19.42304942373100829 ) ) ;
#10322=VECTOR ( 'NONE', #2283, 1000.000000000000000 ) ;
#10325=CARTESIAN_POINT ( 'NONE',  ( -45.81092964171354964, 71.80742102382775727, -12.92463648794852205 ) ) ;
#10330=CIRCLE ( 'NONE', #2107, 2.445500000000003116 ) ;
#10331=CARTESIAN_POINT ( 'NONE',  ( 2.003855453843550460, 35.57695044197526357, -8.044733130177707636 ) ) ;
#10333=CARTESIAN_POINT ( 'NONE',  ( -65.14229033403913149, 38.19691209738603277, 12.92632704043474412 ) ) ;
#10334=CARTESIAN_POINT ( 'NONE',  ( -44.07074648197151845, 61.10275710191199749, -20.11236068975357938 ) ) ;
#10338=CARTESIAN_POINT ( 'NONE',  ( 36.99999999999999289, 64.99999999999998579, 0.000000000000000000 ) ) ;
#10345=CIRCLE ( 'NONE', #7119, 3.000000000000002665 ) ;
#10348=CARTESIAN_POINT ( 'NONE',  ( -62.78770230684006748, 51.59540953287255860, 13.59211127035758260 ) ) ;
#10350=CARTESIAN_POINT ( 'NONE',  ( -7.969360823174009845, 70.58422527244209732, -14.12522777056770629 ) ) ;
#10362=CARTESIAN_POINT ( 'NONE',  ( -30.07727491738399905, 41.06011215405257531, 1.372365971865714407 ) ) ;
#10373=CARTESIAN_POINT ( 'NONE',  ( -12.44324757165961870, 62.02537596287093891, 0.9163237194946400876 ) ) ;
#10380=CARTESIAN_POINT ( 'NONE',  ( -54.88146047731135013, 73.03677976846768161, 10.81065700633557825 ) ) ;
#10384=CARTESIAN_POINT ( 'NONE',  ( -63.06671435217206323, 41.62111505249539078, 16.30162306856191989 ) ) ;
#10387=CARTESIAN_POINT ( 'NONE',  ( 34.00000000000000000, 55.00000000000000000, 0.000000000000000000 ) ) ;
#10389=CARTESIAN_POINT ( 'NONE',  ( -19.00387657603030078, 69.86840152515847535, 14.86901714484747750 ) ) ;
#10391=CARTESIAN_POINT ( 'NONE',  ( -3.522319526695277148, 52.25407378758720256, -20.97954707081091996 ) ) ;
#10392=CARTESIAN_POINT ( 'NONE',  ( 7.872895456215955434, 43.79306672811842560, 8.617525609973794687 ) ) ;
#10398=CARTESIAN_POINT ( 'NONE',  ( -61.71391363462142010, 54.99991449564567603, -0.005034624627165642033 ) ) ;
#10402=CARTESIAN_POINT ( 'NONE',  ( 22.99999999999999645, 76.00000000000000000, 0.000000000000000000 ) ) ;
#10403=CARTESIAN_POINT ( 'NONE',  ( -65.40872037032744402, 46.08084772439340071, 10.86636812464517376 ) ) ;
#10405=CARTESIAN_POINT ( 'NONE',  ( -25.52231952398968673, 42.10919693116569817, 16.77412918608628090 ) ) ;
#10416=CARTESIAN_POINT ( 'NONE',  ( -66.46433446062644634, 41.33748651086542480, 3.672754829735058735 ) ) ;
#10426=CARTESIAN_POINT ( 'NONE',  ( 25.66666666666666430, 61.99999999999997868, 0.000000000000000000 ) ) ;
#10433=CARTESIAN_POINT ( 'NONE',  ( -47.81092963715463640, 71.80394787507084686, -12.92116392654651058 ) ) ;
#10436=CARTESIAN_POINT ( 'NONE',  ( -66.81799029952708224, 34.52069382205590387, 5.503409927558503334 ) ) ;
#10440=CARTESIAN_POINT ( 'NONE',  ( -30.23830917210572267, 50.00000000000000711, 1.120793995806890209E-14 ) ) ;
#10441=CARTESIAN_POINT ( 'NONE',  ( -14.31788144970486165, 59.96719419353341607, -0.6577655422762530568 ) ) ;
#10442=CARTESIAN_POINT ( 'NONE',  ( -32.40407992077046373, 34.08317752212569474, 2.058454929014103651 ) ) ;
#10445=CARTESIAN_POINT ( 'NONE',  ( -10.72515708486913866, 73.59929058593817786, -9.932910085056876781 ) ) ;
#10446=CARTESIAN_POINT ( 'NONE',  ( -2.206240550821941593, 47.95770083149849228, -12.21699568532449121 ) ) ;
#10450=CARTESIAN_POINT ( 'NONE',  ( -67.56971494453328830, 50.00000002031717372, -0.0004507456344833478141 ) ) ;
#10457=CARTESIAN_POINT ( 'NONE',  ( -10.62461255960855233, 60.19719913025998181, -4.710188242643384093 ) ) ;
#10460=CARTESIAN_POINT ( 'NONE',  ( -13.14429486149114013, 76.02373996650987920, 2.745652855075435994 ) ) ;
#10472=CARTESIAN_POINT ( 'NONE',  ( 12.52240408941406535, 44.41801188983610871, 18.37272825892985040 ) ) ;
#10474=CARTESIAN_POINT ( 'NONE',  ( -78.00000000000000000, 54.99999999999999289, 0.000000000000000000 ) ) ;
#10485=CARTESIAN_POINT ( 'NONE',  ( -53.08379927897976813, 60.41024208566564369, 4.439607033037889394 ) ) ;
#10488=EDGE_LOOP ( 'NONE', ( #2037, #8966, #4440, #7061, #10592, #3916 ) ) ;
#10493=LINE ( 'NONE', #7753, #9173 ) ;
#10502=CARTESIAN_POINT ( 'NONE',  ( -43.21475900837984341, 58.08538667521604282, -20.80084980650556759 ) ) ;
#10504=CARTESIAN_POINT ( 'NONE',  ( 4.118574298861553906, 34.19883370460495087, -3.085387377675621767 ) ) ;
#10506=CARTESIAN_POINT ( 'NONE',  ( -44.12197311277270728, 58.40423241926509235, -13.59316381755316350 ) ) ;
#10513=CARTESIAN_POINT ( 'NONE',  ( -66.09273081889568857, 55.00395080879571452, -0.007536095274406174466 ) ) ;
#10516=CARTESIAN_POINT ( 'NONE',  ( -33.08380120443626993, 48.03207042869781418, 0.6864286361564611028 ) ) ;
#10518=CARTESIAN_POINT ( 'NONE',  ( -20.50647613538409075, 59.12524989819403487, 20.69783765389080799 ) ) ;
#10531=CARTESIAN_POINT ( 'NONE',  ( 7.506399388638331338, 34.30832474160909129, 4.109400874309620200 ) ) ;
#10533=AXIS2_PLACEMENT_3D ( 'NONE', #607, #1395, #3361 ) ;
#10537=EDGE_CURVE ( 'NONE', #1675, #2759, #11075, .T. ) ;
#10545=PLANE ( 'NONE',  #6736 ) ;
#10547=CARTESIAN_POINT ( 'NONE',  ( -41.41713581769108998, 57.03123113432517499, -6.697302567478903512 ) ) ;
#10551=VECTOR ( 'NONE', #11388, 1000.000000000000000 ) ;
#10560=CARTESIAN_POINT ( 'NONE',  ( 7.618938171403620174, 55.00878100866180631, 0.0002433764497684456950 ) ) ;
#10564=CARTESIAN_POINT ( 'NONE',  ( -50.14429338685609849, 75.46958046783008456, -5.506903914760000518 ) ) ;
#10566=CARTESIAN_POINT ( 'NONE',  ( 0.9415095817738947659, 38.70554731314401664, -13.38234376684299143 ) ) ;
#10567=CARTESIAN_POINT ( 'NONE',  ( -39.53949924438659025, 47.95754239612929837, -12.21692829552484660 ) ) ;
#10569=CARTESIAN_POINT ( 'NONE',  ( -24.81855061910753690, 54.66933223131182729, 4.999996196634724832 ) ) ;
#10575=CARTESIAN_POINT ( 'NONE',  ( -54.66652844283319723, 61.47673604987254237, 2.683042620825347058 ) ) ;
#10577=CARTESIAN_POINT ( 'NONE',  ( -30.11869220662914159, 34.20731585996448132, 3.085050890631813036 ) ) ;
#10578=CARTESIAN_POINT ( 'NONE',  ( 4.636023424558444184, 34.00634798409771520, 1.031279783234476222 ) ) ;
#10581=EDGE_CURVE ( 'NONE', #1342, #3861, #9590, .T. ) ;
#10582=CARTESIAN_POINT ( 'NONE',  ( 36.99999999999999289, 55.00000000000000000, 0.000000000000000000 ) ) ;
#10588=CARTESIAN_POINT ( 'NONE',  ( 2.274842917244503937, 38.70728229458904934, -13.38060881307704975 ) ) ;
#10592=ORIENTED_EDGE ( 'NONE', *, *, #5968, .F. ) ;
#10600=CARTESIAN_POINT ( 'NONE',  ( -52.20817410683172710, 61.01528383336308536, 3.605005717731896819 ) ) ;
#10608=DIRECTION ( 'NONE',  ( 6.033820786006286457E-17, -1.000000000000000000, 0.000000000000000000 ) ) ;
#10609=CARTESIAN_POINT ( 'NONE',  ( 6.756927758781439586, 54.99032605594245382, -0.0009204374784672792213 ) ) ;
#10615=CARTESIAN_POINT ( 'NONE',  ( -7.929357056070021947, 64.91238717040420170, -18.54984206437098493 ) ) ;
#10617=CARTESIAN_POINT ( 'NONE',  ( -24.52239577716529340, 49.50814072396850918, 20.43329749385727112 ) ) ;
#10618=CARTESIAN_POINT ( 'NONE',  ( -16.20616591473740797, 68.61844237587234829, 3.658903313587498651 ) ) ;
#10626=CARTESIAN_POINT ( 'NONE',  ( 20.31540248889015032, 58.05033696222945139, 3.975385948103875577 ) ) ;
#10627=CARTESIAN_POINT ( 'NONE',  ( -12.08425351220556898, 61.19227081298861037, -3.308756493662277975 ) ) ;
#10629=CARTESIAN_POINT ( 'NONE',  ( 3.929252901860227354, 34.88880312433069264, -6.102315970099479792 ) ) ;
#10640=CARTESIAN_POINT ( 'NONE',  ( 8.058385817489730485, 34.79396711235183659, 6.140502173211014103 ) ) ;
#10646=B_SPLINE_CURVE_WITH_KNOTS ( 'NONE', 3,
 ( #2452, #8866, #4307, #3406, #10704, #2517, #6181, #5330, #999, #2689, #3701, #3821, #5564, #6592, #7365, #10990, #10940, #1779, #4600, #92, #10878, #11834, #4658, #873, #1896, #7254, #5687, #935, #8311, #5504, #1958, #4546, #1057, #5627, #10222, #4781 ),
 .UNSPECIFIED., .F., .F.,
 ( 4, 2, 2, 2, 2, 2, 2, 2, 2, 2, 2, 2, 2, 2, 2, 2, 2, 4 ),
 ( 0.000000000000000000, 0.001517583048112853628, 0.003035166096225707256, 0.004552749144338561101, 0.006070332192451414512, 0.007587915240564267055, 0.008346706764620690291, 0.009105498288677110058, 0.01214066438490281168, 0.01365824743301567550, 0.01517583048112853931, 0.01593462200518497990, 0.01669341352924142222, 0.01821099657735429297, 0.01972857962546716026, 0.02124616267358003102, 0.02276374572169290525, 0.02428132876980577601 ),
 .UNSPECIFIED. ) ;
#10647=CARTESIAN_POINT ( 'NONE',  ( 34.00000000000000000, 55.00000000000000000, 0.000000000000000000 ) ) ;
#10648=CARTESIAN_POINT ( 'NONE',  ( -32.40407992077046373, 34.08317752212569474, 2.058454929014103651 ) ) ;
#10652=CARTESIAN_POINT ( 'NONE',  ( -71.09399662003431786, 50.00000004634800632, -0.0006807936302138478625 ) ) ;
#10658=CARTESIAN_POINT ( 'NONE',  ( -29.75046914791206731, 48.03518065199703813, 0.6863338727569227027 ) ) ;
#10671=CARTESIAN_POINT ( 'NONE',  ( -3.170201962785300420, 54.99752259272338506, 0.005286603947392433563 ) ) ;
#10674=CARTESIAN_POINT ( 'NONE',  ( -27.12855804074951394, 50.66807883178916683, 2.502284342222150570 ) ) ;
#10678=CARTESIAN_POINT ( 'NONE',  ( -40.49360049774279702, 50.89060478259270326, -20.69231637581390260 ) ) ;
#10679=CARTESIAN_POINT ( 'NONE',  ( -40.92871871552156193, 50.90608857496490458, -13.47236005574864492 ) ) ;
#10688=EDGE_CURVE ( 'NONE', #4223, #3357, #3218, .T. ) ;
#10691=CARTESIAN_POINT ( 'NONE',  ( 21.47836779243698402, 58.76591268667433354, 3.305356925373596155 ) ) ;
#10692=CARTESIAN_POINT ( 'NONE',  ( -36.77654997417609906, 48.86760992094172451, -3.531900520213358430 ) ) ;
#10696=CARTESIAN_POINT ( 'NONE',  ( -60.73530621856283318, 48.89645762657089278, 20.10868697360108115 ) ) ;
#10697=FACE_OUTER_BOUND ( 'NONE', #3999, .T. ) ;
#10704=CARTESIAN_POINT ( 'NONE',  ( -65.62689358872800938, 50.25421578100692699, 1.608180852589480070 ) ) ;
#10705=CARTESIAN_POINT ( 'NONE',  ( 4.003855478097921861, 35.57747403031575573, -8.044509115018048107 ) ) ;
#10708=CARTESIAN_POINT ( 'NONE',  ( -54.37477180893560558, 59.74454033230625782, 1.611245227688210324 ) ) ;
#10711=CARTESIAN_POINT ( 'NONE',  ( -56.32961277634869646, 69.86611656190129338, 14.86520567151240080 ) ) ;
#10719=CARTESIAN_POINT ( 'NONE',  ( -41.12525411544546472, 56.70070297179961472, -6.793461455911497637 ) ) ;
#10721=FACE_OUTER_BOUND ( 'NONE', #6843, .T. ) ;
#10725=AXIS2_PLACEMENT_3D ( 'NONE', #10474, #11427, #2340 ) ;
#10733=CARTESIAN_POINT ( 'NONE',  ( 11.24060940615075488, 54.98030487590998661, 0.01734873002535425313 ) ) ;
#10739=CARTESIAN_POINT ( 'NONE',  ( -70.34104699118842063, 33.99562393659818582, 0.006612473344882202446 ) ) ;
#10741=CARTESIAN_POINT ( 'NONE',  ( -54.21479381498274108, 73.03707320332732422, 10.81077985938301822 ) ) ;
#10742=CARTESIAN_POINT ( 'NONE',  ( -46.73803912521919557, 63.91895867764292660, -10.86094668994167023 ) ) ;
#10746=DIRECTION ( 'NONE',  ( 0.000000000000000000, 0.000000000000000000, 1.000000000000000000 ) ) ;
#10749=CARTESIAN_POINT ( 'NONE',  ( 10.98755190560986961, 51.02739634541043046, 3.053971085653802486 ) ) ;
#10750=CARTESIAN_POINT ( 'NONE',  ( 1.576338153721813740, 55.00586181284610632, 0.002877765224681509519 ) ) ;
#10752=CARTESIAN_POINT ( 'NONE',  ( -11.47759590222061021, 75.47256375259368610, -5.508258824058441583 ) ) ;
#10753=CARTESIAN_POINT ( 'NONE',  ( -32.99614454614441428, 33.97685596767119165, 0.0005149883856687357403 ) ) ;
#10758=ORIENTED_EDGE ( 'NONE', *, *, #5953, .T. ) ;
#10762=CARTESIAN_POINT ( 'NONE',  ( -59.88037020503378471, 51.91452991566635689, 20.80113349088246011 ) ) ;
#10770=CARTESIAN_POINT ( 'NONE',  ( 13.29588712016585106, 55.33163179650340169, 5.000002229370401174 ) ) ;
#10773=EDGE_LOOP ( 'NONE', ( #7466, #4056, #10102, #10864 ) ) ;
#10777=CARTESIAN_POINT ( 'NONE',  ( 19.12717080529655078, 62.03996031863259475, 12.21087854330282951 ) ) ;
#10789=CARTESIAN_POINT ( 'NONE',  ( 7.335481199539121810, 54.99686737186916474, -0.0001706956380964400033 ) ) ;
#10792=ORIENTED_EDGE ( 'NONE', *, *, #6593, .T. ) ;
#10796=CARTESIAN_POINT ( 'NONE',  ( -22.39182375099971267, 57.05917196451265028, 20.98466401600494891 ) ) ;
#10805=ADVANCED_FACE ( 'NONE', ( #9046 ), #11609, .F. ) ;
#10806=CARTESIAN_POINT ( 'NONE',  ( 9.573972992054704534, 54.99220333846943021, 0.01448963470816768892 ) ) ;
#10809=CARTESIAN_POINT ( 'NONE',  ( 13.47757237172695000, 49.50866688550052430, 20.43174547745228864 ) ) ;
#10810=CARTESIAN_POINT ( 'NONE',  ( -39.18898618735786243, 44.43394377878069434, -18.33326528472845141 ) ) ;
#10821=CARTESIAN_POINT ( 'NONE',  ( -66.81799029952708224, 34.52069382205590387, 5.503409927558503334 ) ) ;
#10824=PRODUCT ( 'Internal Tapered Feed Screw Auger', 'Internal Tapered Feed Screw Auger', '', ( #2829 ) ) ;
#10825=CONICAL_SURFACE ( 'NONE', #876, 2.999999999999995559, 0.7853981633974420618 ) ;
#10826=CARTESIAN_POINT ( 'NONE',  ( -63.31773346265211444, 53.70568493644218933, 4.840560537982487865 ) ) ;
#10827=B_SPLINE_CURVE_WITH_KNOTS ( 'NONE', 3,
 ( #4517, #1700, #10011, #732, #9015, #1806, #9960, #5474, #9122, #8214, #2644, #1912, #9165, #951, #2708, #6310, #6254, #5346, #774, #10952, #8272, #1741, #9998, #8999, #10837, #4450, #11849, #11679, #3539, #8103, #46, #5405, #8041, #4617, #3714, #9882 ),
 .UNSPECIFIED., .F., .F.,
 ( 4, 2, 2, 2, 2, 2, 2, 2, 2, 2, 2, 2, 2, 2, 2, 2, 2, 4 ),
 ( 0.07284642870127019942, 0.07360525742480880651, 0.07436408614834741360, 0.07588174359542464165, 0.07739940104250185582, 0.07891705848957906999, 0.08043471593665629804, 0.08195237338373351221, 0.08347003083081072639, 0.08498768827788795444, 0.08574651700142656152, 0.08650534572496516861, 0.08802300317204239666, 0.08954066061911961083, 0.09105831806619682500, 0.09257597551327405305, 0.09409363296035126722, 0.09712894785450570945 ),
 .UNSPECIFIED. ) ;
#10828=ORIENTED_EDGE ( 'NONE', *, *, #8050, .T. ) ;
#10830=CARTESIAN_POINT ( 'NONE',  ( 17.95684494300012801, 58.76662442904990513, 3.304478729834980921 ) ) ;
#10837=CARTESIAN_POINT ( 'NONE',  ( -0.2902744515997993657, 53.38936837472795816, -4.744839395679999683 ) ) ;
#10839=CARTESIAN_POINT ( 'NONE',  ( 6.664798253476140744, 40.98022014747188990, -0.0003427094624634590900 ) ) ;
#10847=ADVANCED_FACE ( 'NONE', ( #6303 ), #5397, .T. ) ;
#10852=CARTESIAN_POINT ( 'NONE',  ( -39.33118544708877096, 55.00017070458616786, -0.003132656074481668385 ) ) ;
#10856=CARTESIAN_POINT ( 'NONE',  ( -25.95462006380511966, 51.23402121196087933, 3.305273135093794501 ) ) ;
#10859=CARTESIAN_POINT ( 'NONE',  ( -29.69731012496106359, 35.99954121986550604, 8.986476355089152435 ) ) ;
#10863=CARTESIAN_POINT ( 'NONE',  ( 2.826857198123298165, 37.44742646213195769, -11.71858918393001225 ) ) ;
#10864=ORIENTED_EDGE ( 'NONE', *, *, #365, .T. ) ;
#10866=CARTESIAN_POINT ( 'NONE',  ( 0.9978688846961245584, 55.00160005685901865, 0.0008981051542724318056 ) ) ;
#10868=CARTESIAN_POINT ( 'NONE',  ( 6.839732782626861685, 34.30800418419381259, 4.109398041371060017 ) ) ;
#10869=CARTESIAN_POINT ( 'NONE',  ( -7.030643242133587378, 62.08114452727563304, -19.79025909736091648 ) ) ;
#10876=FACE_OUTER_BOUND ( 'NONE', #11478, .T. ) ;
#10877=CARTESIAN_POINT ( 'NONE',  ( -20.87154949818722116, 55.00167759324021688, 0.002033656601463836207 ) ) ;
#10878=CARTESIAN_POINT ( 'NONE',  ( -56.29331228730723069, 56.60826288146544272, 4.745686675311040048 ) ) ;
#10884=CARTESIAN_POINT ( 'NONE',  ( -67.20012888935585238, 51.02918010271523030, 3.055874726862140900 ) ) ;
#10886=VERTEX_POINT ( 'NONE', #9935 ) ;
#10887=DIRECTION ( 'NONE',  ( 0.000000000000000000, 1.000000000000000000, 0.000000000000000000 ) ) ;
#10898=CARTESIAN_POINT ( 'NONE',  ( -26.59538538879835556, 44.11636033083960484, 8.941403297748980350 ) ) ;
#10911=CARTESIAN_POINT ( 'NONE',  ( -30.00213106679868957, 55.00296086862838507, 0.0002306145982448079112 ) ) ;
#10915=ORIENTED_EDGE ( 'NONE', *, *, #197, .T. ) ;
#10916=CARTESIAN_POINT ( 'NONE',  ( -63.63584090060282961, 46.00639722032484968, 19.01118640546643590 ) ) ;
#10917=EDGE_CURVE ( 'NONE', #4670, #7593, #1842, .T. ) ;
#10919=CARTESIAN_POINT ( 'NONE',  ( 1.697306494461763959, 35.98764835359665426, -8.991780390316415961 ) ) ;
#10925=CARTESIAN_POINT ( 'NONE',  ( -17.88142570751413274, 67.52739394234649239, 16.89079266652326439 ) ) ;
#10929=CARTESIAN_POINT ( 'NONE',  ( -10.66879778189107419, 54.99855794386581209, 0.001134569799796503100 ) ) ;
#10930=ORIENTED_EDGE ( 'NONE', *, *, #11161, .F. ) ;
#10931=CARTESIAN_POINT ( 'NONE',  ( -59.67156972769491574, 55.00060627355243525, 21.02858942331178227 ) ) ;
#10932=CARTESIAN_POINT ( 'NONE',  ( -19.59602372284622618, 68.34451306940553650, 16.25656885606184332 ) ) ;
#10934=PLANE ( 'NONE',  #6211 ) ;
#10939=CARTESIAN_POINT ( 'NONE',  ( -53.83687749268464984, 54.99647651120280045, -0.001734407420701496736 ) ) ;
#10940=CARTESIAN_POINT ( 'NONE',  ( -59.02007697189144153, 54.33745946848893738, 5.000024639461678966 ) ) ;
#10946=CARTESIAN_POINT ( 'NONE',  ( 16.01486940960983674, 57.50823208304175438, 4.337747975045839866 ) ) ;
#10952=CARTESIAN_POINT ( 'NONE',  ( -2.043570261588242953, 54.83463289114614270, -4.999998501150977326 ) ) ;
#10953=CARTESIAN_POINT ( 'NONE',  ( -20.73803862786483165, 56.37319242487460258, 13.98159745988486868 ) ) ;
#10962=CARTESIAN_POINT ( 'NONE',  ( -58.87201974314975672, 55.00020036712756877, 0.003823789621534544932 ) ) ;
#10964=CARTESIAN_POINT ( 'NONE',  ( 36.99999999999999289, 55.00000000000000000, 0.000000000000000000 ) ) ;
#10969=ORIENTED_EDGE ( 'NONE', *, *, #2171, .T. ) ;
#10970=CARTESIAN_POINT ( 'NONE',  ( 21.47754340280339136, 75.43473409906381733, 5.492671141289128478 ) ) ;
#10974=CARTESIAN_POINT ( 'NONE',  ( -5.337209886265139147, 63.04750289227570192, -19.42727033598380970 ) ) ;
#10979=CARTESIAN_POINT ( 'NONE',  ( -58.16650030231640045, 58.91145824815324517, 5.848851387972111127 ) ) ;
#10981=CARTESIAN_POINT ( 'NONE',  ( -41.00387659642365179, 55.00043089085527726, -21.02791246669550773 ) ) ;
#10982=CARTESIAN_POINT ( 'NONE',  ( -23.05849041873830885, 57.05917197429855037, 20.98589082339331569 ) ) ;
#10988=DIRECTION ( 'NONE',  ( 0.000000000000000000, 1.000000000000000000, 0.000000000000000000 ) ) ;
#10989=CARTESIAN_POINT ( 'NONE',  ( -39.42605725089504176, 54.98959656231615156, -0.01274862175783714538 ) ) ;
#10990=CARTESIAN_POINT ( 'NONE',  ( -59.79376487574317167, 53.69725619367564207, 4.871814158559260477 ) ) ;
#10992=CARTESIAN_POINT ( 'NONE',  ( 36.99999999999999289, 55.00000000000000000, 0.000000000000000000 ) ) ;
#10994=EDGE_LOOP ( 'NONE', ( #3661, #2455, #10758, #3565 ) ) ;
#10997=CARTESIAN_POINT ( 'NONE',  ( -28.71241679207687625, 51.69383968972351795, 3.765155372993232330 ) ) ;
#11006=CARTESIAN_POINT ( 'NONE',  ( -7.331473370266870404, 64.90913857603797510, -9.909739041900611056 ) ) ;
#11016=CARTESIAN_POINT ( 'NONE',  ( -21.42602701979682323, 54.99834091475071318, 0.02619292028802366196 ) ) ;
#11023=CARTESIAN_POINT ( 'NONE',  ( 8.071484979291650319, 50.06510116776722441, 0.8205671114678182443 ) ) ;
#11028=CARTESIAN_POINT ( 'NONE',  ( 15.18896243380506306, 60.50666922109576262, 20.46968130491651650 ) ) ;
#11032=CARTESIAN_POINT ( 'NONE',  ( -41.21475901749523274, 58.08538884819615333, -20.80179922188357011 ) ) ;
#11034=CARTESIAN_POINT ( 'NONE',  ( -38.60828084422895046, 48.85949782923615459, -20.20603288453101243 ) ) ;
#11038=CARTESIAN_POINT ( 'NONE',  ( 21.47754340280339136, 75.43473409906381733, 5.492671141289128478 ) ) ;
#11041=ADVANCED_FACE ( 'NONE', ( #7551 ), #8724, .T. ) ;
#11042=CARTESIAN_POINT ( 'NONE',  ( -52.67050196621227798, 74.42705245932049252, 8.047455632081089050 ) ) ;
#11044=CARTESIAN_POINT ( 'NONE',  ( -42.92935705524211443, 57.05913440163546113, -20.93112575922673102 ) ) ;
#11052=CARTESIAN_POINT ( 'NONE',  ( -57.33538960692911957, 54.99887155840742992, -0.001353544291193513891 ) ) ;
#11053=CARTESIAN_POINT ( 'NONE',  ( -36.85275351908241959, 52.78708903700569977, -4.486665150141578629 ) ) ;
#11058=CARTESIAN_POINT ( 'NONE',  ( -61.33571477330379196, 55.00015097948840292, 14.01955991042104444 ) ) ;
#11072=CARTESIAN_POINT ( 'NONE',  ( -44.07137245399455594, 63.91548889941181244, -10.85747687929244165 ) ) ;
#11075=LINE ( 'NONE', #2887, #143 ) ;
#11083=CARTESIAN_POINT ( 'NONE',  ( 17.10991510816216987, 55.91632096216925163, 6.974641958105268991 ) ) ;
#11090=CARTESIAN_POINT ( 'NONE',  ( -19.88142569839470042, 67.52672413929985851, 16.89011978890229315 ) ) ;
#11094=CARTESIAN_POINT ( 'NONE',  ( -18.73741402030934111, 64.90551912913463184, 18.53518525054827393 ) ) ;
#11095=AXIS2_PLACEMENT_3D ( 'NONE', #7252, #4543, #4431 ) ;
#11096=FACE_OUTER_BOUND ( 'NONE', #9727, .T. ) ;
#11100=CARTESIAN_POINT ( 'NONE',  ( -1.855729112296511385, 44.43418165317581980, -18.33336562707187412 ) ) ;
#11102=CARTESIAN_POINT ( 'NONE',  ( -48.81096005563045992, 75.47260553545579853, -5.508156592082438685 ) ) ;
#11104=CARTESIAN_POINT ( 'NONE',  ( -48.52239103406665066, 73.33336493528216238, -10.56581381373428208 ) ) ;
#11106=DIRECTION ( 'NONE',  ( -1.000000000000000000, -6.033820786006286457E-17, 0.000000000000000000 ) ) ;
#11111=CARTESIAN_POINT ( 'NONE',  ( -53.23625741230951292, 55.01228365700361422, 0.001247673927939117831 ) ) ;
#11112=CARTESIAN_POINT ( 'NONE',  ( -46.18628267998333570, 59.48674120129327747, -2.212764751379967976 ) ) ;
#11117=CARTESIAN_POINT ( 'NONE',  ( -55.21148394789464220, 67.02529821378587371, 7.207524229417598072 ) ) ;
#11123=B_SPLINE_CURVE_WITH_KNOTS ( 'NONE', 3,
 ( #10440, #8841, #620, #7941, #11576, #3377, #7054, #10674, #3616, #1867, #10856, #3441, #7341, #9068, #9182, #5364, #1755, #5534, #792, #970, #1635, #846, #2604, #8172, #11812, #4408, #11633, #8960, #8059, #8, #9904, #7284, #6210, #3559, #7230, #8231, #2662, #6437 ),
 .UNSPECIFIED., .F., .F.,
 ( 4, 2, 2, 2, 2, 2, 2, 2, 2, 2, 2, 2, 2, 2, 2, 2, 2, 2, 4 ),
 ( 0.04856354657319568446, 0.05008122670620035466, 0.05159890683920503179, 0.05235774690570735995, 0.05311658697220968811, 0.05463426710521434443, 0.05615194723821900769, 0.05766962737122366400, 0.05918730750422832032, 0.06070498763723297664, 0.06146382770373530480, 0.06222266777023762602, 0.06374034790324227540, 0.06525802803624693171, 0.06677570816925158803, 0.06829338830225623047, 0.06981106843526088679, 0.07132874856826554311, 0.07284642870127019942 ),
 .UNSPECIFIED. ) ;
#11130=CARTESIAN_POINT ( 'NONE',  ( -49.92872185120336326, 69.01842773188042202, 1.373364986375345875 ) ) ;
#11139=CARTESIAN_POINT ( 'NONE',  ( -2.915823261801936628, 55.68730727514731171, -7.019035972284535241 ) ) ;
#11141=DIRECTION ( 'NONE',  ( -1.000000000000000000, -0.000000000000000000, -0.000000000000000000 ) ) ;
#11147=CARTESIAN_POINT ( 'NONE',  ( -7.929357056070021947, 64.91238717040420170, -18.54984206437098493 ) ) ;
#11150=CARTESIAN_POINT ( 'NONE',  ( -68.34104732181950226, 33.99448141944334623, 0.006743540747238889813 ) ) ;
#11151=CARTESIAN_POINT ( 'NONE',  ( -42.07074724807011989, 61.10209548959944215, -20.11061483308460751 ) ) ;
#11156=DIRECTION ( 'NONE',  ( -1.000000000000000000, -0.000000000000000000, -0.000000000000000000 ) ) ;
#11158=CARTESIAN_POINT ( 'NONE',  ( -17.67054322722435700, 69.86867477976171870, 14.86928418406260910 ) ) ;
#11159=CARTESIAN_POINT ( 'NONE',  ( 12.53956257875718805, 53.16901327126123533, 14.01800940675507867 ) ) ;
#11161=EDGE_CURVE ( 'NONE', #1442, #8109, #7709, .T. ) ;
#11164=ORIENTED_EDGE ( 'NONE', *, *, #349, .F. ) ;
#11169=STYLED_ITEM ( 'NONE', ( #4586 ), #2413 ) ;
#11172=CARTESIAN_POINT ( 'NONE',  ( -57.83638956477260251, 62.82127934421545490, 11.69590706508775213 ) ) ;
#11174=CARTESIAN_POINT ( 'NONE',  ( 25.00000000000000000, 76.00000000000000000, 0.000000000000000000 ) ) ;
#11187=CARTESIAN_POINT ( 'NONE',  ( -40.00186843037597129, 55.00034269701549761, -14.01977987948117921 ) ) ;
#11199=CARTESIAN_POINT ( 'NONE',  ( -39.20651884422274946, 51.94919883060119048, -3.974814712047955556 ) ) ;
#11201=CARTESIAN_POINT ( 'NONE',  ( 17.89001317236136757, 56.84184411483420263, 6.841298196563591283 ) ) ;
#11210=CARTESIAN_POINT ( 'NONE',  ( -50.85567158358731632, 75.98119253013058483, -2.745941642920928683 ) ) ;
#11220=DIRECTION ( 'NONE',  ( -0.000000000000000000, -0.000000000000000000, 1.000000000000000000 ) ) ;
#11221=CARTESIAN_POINT ( 'NONE',  ( 12.85570563148687739, 52.25434904275299175, 21.01882863504484789 ) ) ;
#11223=CARTESIAN_POINT ( 'NONE',  ( 13.52237229673245089, 52.25434890037524127, 21.02046579585209329 ) ) ;
#11225=CARTESIAN_POINT ( 'NONE',  ( 3.410516172888891084, 41.04393794207129531, -1.373024938261769856 ) ) ;
#11235=CARTESIAN_POINT ( 'NONE',  ( -61.92257069291975569, 53.62718127820116365, 13.95588266757517815 ) ) ;
#11239=DIRECTION ( 'NONE',  ( -1.000000000000000000, -0.000000000000000000, -0.000000000000000000 ) ) ;
#11248=CARTESIAN_POINT ( 'NONE',  ( 18.81101721030213625, 65.56418867429738384, 18.32872549916029925 ) ) ;
#11259=CARTESIAN_POINT ( 'NONE',  ( -46.99165357442934976, 58.05298380892439525, -3.973364261919617224 ) ) ;
#11262=CARTESIAN_POINT ( 'NONE',  ( -7.000135551824203439, 59.95344092836027272, -4.953904230404519105 ) ) ;
#11270=CARTESIAN_POINT ( 'NONE',  ( -26.81096152405270061, 44.41979049410412017, 18.36814973051028588 ) ) ;
#11275=CARTESIAN_POINT ( 'NONE',  ( -59.88037020503378471, 51.91452991566635689, 20.80113349088246011 ) ) ;
#11281=CARTESIAN_POINT ( 'NONE',  ( 0.2637464422577515122, 50.75252801053527207, -2.643076731290110448 ) ) ;
#11283=CARTESIAN_POINT ( 'NONE',  ( -10.83980928483403794, 72.54296691076741865, -11.73126556815853760 ) ) ;
#11285=CARTESIAN_POINT ( 'NONE',  ( 5.302689875203906666, 34.00688940836099050, 1.031260791178478797 ) ) ;
#11286=CARTESIAN_POINT ( 'NONE',  ( -54.59603348275399526, 73.54984634329692028, 9.912388241271610667 ) ) ;
#11289=UNCERTAINTY_MEASURE_WITH_UNIT (LENGTH_MEASURE( 1.000000000000000082E-05 ), #5611, 'distance_accuracy_value', 'NONE');
#11300=CARTESIAN_POINT ( 'NONE',  ( -8.582943931441322505, 58.30613956700960898, -6.186730322951330407 ) ) ;
#11302=CARTESIAN_POINT ( 'NONE',  ( -24.81096152833125856, 44.41791055217656492, 18.37268719335390443 ) ) ;
#11304=CARTESIAN_POINT ( 'NONE',  ( 53.00000000000000000, 51.46446609406726935, 3.535533905932731091 ) ) ;
#11310=AXIS2_PLACEMENT_3D ( 'NONE', #10992, #9930, #11836 ) ;
#11311=AXIS2_PLACEMENT_3D ( 'NONE', #8954, #7444, #6206 ) ;
#11313=CARTESIAN_POINT ( 'NONE',  ( -53.12201214189175147, 66.25487413167280693, 8.346098093582366317 ) ) ;
#11321=CARTESIAN_POINT ( 'NONE',  ( -43.87781470623360747, 55.65760560131963786, -4.959288383363730901 ) ) ;
#11323=CARTESIAN_POINT ( 'NONE',  ( -10.89008531556037163, 61.97464205804329396, -0.9163204594661494840 ) ) ;
#11331=CARTESIAN_POINT ( 'NONE',  ( -25.18906244525692983, 49.50751464484449826, 20.43480895838654376 ) ) ;
#11334=CARTESIAN_POINT ( 'NONE',  ( -44.39182476880109363, 68.38060868816502591, -16.29271878486493463 ) ) ;
#11341=CARTESIAN_POINT ( 'NONE',  ( -8.214759031591983174, 65.81066618478850216, -18.03675305545087681 ) ) ;
#11343=CARTESIAN_POINT ( 'NONE',  ( -67.48465754769044622, 34.52249208990708951, 5.502706378135331811 ) ) ;
#11344=CARTESIAN_POINT ( 'NONE',  ( -18.16357859702436173, 66.69092602918284740, 7.816436488534476368 ) ) ;
#11349=EDGE_LOOP ( 'NONE', ( #764, #11616, #8823, #3632 ) ) ;
#11355=CARTESIAN_POINT ( 'NONE',  ( -37.55675198932200232, 49.41446278833375771, -4.289664455798599896 ) ) ;
#11358=CARTESIAN_POINT ( 'NONE',  ( -34.14426257084027583, 36.62727174719971401, -10.58198811264723282 ) ) ;
#11368=CARTESIAN_POINT ( 'NONE',  ( -16.69731055678936826, 70.57278980777935828, 14.11442052818484783 ) ) ;
#11372=( GEOMETRIC_REPRESENTATION_CONTEXT ( 3 ) GLOBAL_UNCERTAINTY_ASSIGNED_CONTEXT ( ( #9333 ) ) GLOBAL_UNIT_ASSIGNED_CONTEXT ( ( #2744, #7248, #10153 ) ) REPRESENTATION_CONTEXT ( 'NONE', 'WORKASPACE' ) );
#11375=CARTESIAN_POINT ( 'NONE',  ( 36.99999999999999289, 50.00000000000001421, 6.123233995736750505E-16 ) ) ;
#11378=CARTESIAN_POINT ( 'NONE',  ( -40.54150824691468102, 56.02863368430912772, -6.936948454549333398 ) ) ;
#11382=B_SPLINE_SURFACE_WITH_KNOTS ( 'NONE', 3, 3, ( 
 ( #617, #8891, #8836, #672, #4343, #3258, #4279, #1578, #3373, #3498, #11448, #3435, #11630, #10733, #497, #729, #6930, #10560, #10789, #10609, #5182, #7108, #2418, #9781, #7049, #6089, #2360, #9612, #2541, #7164, #1404, #6207, #10671, #4219, #5069, #8775, #3320, #7993, #9721, #9841, #1632, #6147, #8714, #7881, #8054, #11697, #5244, #4156, #7817, #6031, #11512, #9666, #1464, #5126, #5300, #553, #1518, #7938, #2482, #11016, #4462, #9118, #3, #2659, #1753, #1695, #3555, #5359, #4631, #9237, #9899, #10911, #8114, #1025, #901, #2720, #6495, #1926, #6381, #9065, #842, #2773, #10852, #3673, #11749, #4573, #6267, #10009, #7225, #5471, #788, #966, #6326, #59, #8282, #9956, #8227, #3725, #5417, #6433, #9010, #4513, #3787, #121, #7389, #10065, #9178, #4685, #8168, #7336, #2599, #2828, #10962, #8337, #11809, #10124, #7456, #3613, #1864, #7280, #1803, #5599, #5530, #5720 ),
 ( #10426, #7631, #2167, #2955, #8590, #10310, #9290, #11201, #11083, #9355, #7689, #4087, #6619, #5897, #4874, #9417, #2894, #2228, #2045, #4995, #186, #9540, #366, #1331, #4751, #6742, #6563, #3972, #1144, #10193, #3073, #11139, #2106, #4031, #1266, #1086, #5781, #4935, #8403, #11262, #1985, #3853, #428, #8647, #11323, #10373, #5837, #5653, #7518, #1208, #10248, #3132, #8524, #4814, #8469, #6799, #246, #3910, #9477, #7574, #3011, #6680, #308, #2350, #6019, #9601, #3360, #1508, #7096, #4269, #10658, #11438, #5233, #6975, #5962, #7868, #7747, #9654, #4325, #717, #3247, #2531, #5170, #6078, #11378, #10719, #10547, #1620, #8703, #6197, #8881, #9831, #1394, #7036, #3188, #606, #1449, #6861, #11557, #7806, #10600, #5114, #10485, #8762, #543, #2468, #4207, #6134, #1568, #7926, #2289, #11500, #5285, #8939, #9769, #5056, #486, #4143, #3308, #6916, #2404, #9712, #659, #8824 ),
 ( #7982, #11619, #3422, #7327, #775, #3716, #10777, #7214, #9054, #7154, #9226, #11680, #6424, #5406, #4389, #1853, #2590, #3540, #10839, #9000, #1794, #3489, #4503, #4618, #6373, #7379, #8156, #2709, #9999, #9945, #8104, #890, #11850, #6256, #9884, #5520, #4564, #830, #3603, #11006, #11798, #2819, #6486, #5461, #1679, #7268, #5348, #2645, #6311, #10054, #8273, #2763, #10115, #9109, #8216, #1913, #5583, #3663, #10953, #4451, #8042, #11740, #1742, #10898, #9167, #952, #47, #3061, #2031, #5883, #10362, #3777, #173, #3841, #5643, #10299, #108, #1133, #1252, #3000, #4020, #4800, #11187, #6670, #6610, #4739, #9405, #8327, #1013, #7445, #11072, #7677, #2883, #8458, #7508, #11130, #5707, #4922, #6730, #4674, #5828, #11313, #6550, #295, #2157, #237, #10181, #2095, #8575, #353, #2217, #1974, #9467, #3122, #5767, #9279, #1071, #8393, #7563, #2943, #6787, #10416, #1199, #3958 ),
 ( #3900, #8513, #4864, #10237, #9344, #7620, #11248, #2454, #4078, #647, #6848, #10472, #2518, #2339, #8747, #10640, #10531, #1497, #6963, #6008, #2272, #9527, #6119, #10705, #7080, #9754, #10588, #9641, #4131, #1315, #4309, #7967, #5948, #531, #4984, #3346, #2389, #3408, #473, #7018, #8634, #11602, #8811, #7793, #1437, #1551, #7854, #11426, #3233, #11368, #5156, #3294, #8867, #6065, #588, #1384, #5218, #4194, #7737, #5102, #415, #6903, #3177, #9586, #5045, #8691, #9699, #11482, #4254, #7913, #11542, #203, #7140, #9311, #7475, #5670, #11665, #1943, #1606, #11034, #8091, #5273, #10141, #6240, #5548, #4434, #11151, #8983, #3525, #1039, #2629, #9250, #137, #6513, #6182, #11726, #1100, #4763, #5612, #9814, #8921, #8419, #7196, #3870, #702, #4375, #4705, #7529, #8026, #3475, #1999, #2911, #10762, #984, #3741, #9869, #5332, #2573, #1663, #759, #8357, #10821, #6450, #10081 ) ),
 .UNSPECIFIED., .F., .F., .F.,
 ( 4, 4 ),
 ( 4, 2, 2, 2, 2, 2, 2, 2, 2, 2, 2, 2, 2, 2, 2, 2, 2, 2, 2, 2, 2, 2, 2, 2, 2, 2, 2, 2, 2, 2, 2, 2, 2, 2, 2, 2, 2, 2, 2, 2, 2, 2, 2, 2, 2, 2, 2, 2, 2, 2, 2, 2, 2, 2, 2, 2, 2, 2, 2, 2, 2, 4 ),
 ( 0.000000000000000000, 1.000000000000000000 ),
 ( 0.000000000000000000, 0.02499977550252127645, 0.04999988577693819519, 0.07499999605135511394, 0.09999999831535408279, 0.1250000005793530378, 0.1500000028441162425, 0.1750000051088794195, 0.1937500039558066045, 0.2031250033792701970, 0.2125000028027338173, 0.2218750022261974375, 0.2312500016496610300, 0.2500000004965882150, 0.2750000027613288545, 0.3000000050260694384, 0.3187500038730080032, 0.3281250032964772578, 0.3375000027199465125, 0.3468750021434158226, 0.3562500015668850772, 0.3750000004138236420, 0.4000000026785641705, 0.4250000049433046989, 0.4437500037902432082, 0.4531250032137125183, 0.4625000026371817730, 0.4718750020606510276, 0.4812500014841203377, 0.5000000003310588470, 0.5250000025957997085, 0.5500000048605405700, 0.5687500037074788573, 0.5781250031309480564, 0.5875000025544172555, 0.5968750019778864546, 0.6062500014013556537, 0.6250000002482940520, 0.6500000025128280789, 0.6750000047773621059, 0.6937500036244039769, 0.7031250030479249125, 0.7125000024714458480, 0.7218750018949667835, 0.7312500013184877190, 0.7500000001655295900, 0.7750000023794885173, 0.8000000045934475557, 0.8187500034657768655, 0.8281250029019414649, 0.8375000023381060643, 0.8468750017742707747, 0.8562500012104353742, 0.8750000000827646840, 0.8937502654913498379, 0.9031253981956424148, 0.9125005308999349918, 0.9218756636042275687, 0.9312507963085201457, 0.9500010617171052996, 0.9750005308585526498, 1.000000000000000000 ),
 .UNSPECIFIED. ) ;
#11386=ORIENTED_EDGE ( 'NONE', *, *, #6255, .T. ) ;
#11388=DIRECTION ( 'NONE',  ( -1.000000000000000000, -0.000000000000000000, -0.000000000000000000 ) ) ;
#11393=CARTESIAN_POINT ( 'NONE',  ( -34.72515708538001888, 34.82355399787605421, -6.128525890628534256 ) ) ;
#11395=CARTESIAN_POINT ( 'NONE',  ( -63.73338128346249221, 41.62050876239434416, 16.30218879057518322 ) ) ;
#11396=CARTESIAN_POINT ( 'NONE',  ( -31.87813363146436885, 41.40035587688806373, 3.406667234184215243 ) ) ;
#11399=CARTESIAN_POINT ( 'NONE',  ( -17.81440531450395071, 59.49424450570884204, 2.215684812588340158 ) ) ;
#11408=CIRCLE ( 'NONE', #6090, 3.000000000000002665 ) ;
#11409=DIRECTION ( 'NONE',  ( -1.000000000000000000, -0.000000000000000000, -0.000000000000000000 ) ) ;
#11410=CARTESIAN_POINT ( 'NONE',  ( -18.50022343123301027, 60.84416894878899740, 3.906748298023257071 ) ) ;
#11411=VERTEX_POINT ( 'NONE', #7477 ) ;
#11412=CARTESIAN_POINT ( 'NONE',  ( -19.32947785509334082, 63.04547287423799418, 19.42212676744230393 ) ) ;
#11413=CARTESIAN_POINT ( 'NONE',  ( 22.18771278451687579, 76.01886845420673922, 2.750080521686579793 ) ) ;
#11414=DIRECTION ( 'NONE',  ( -0.000000000000000000, 0.000000000000000000, 1.000000000000000000 ) ) ;
#11420=VERTEX_POINT ( 'NONE', #3872 ) ;
#11425=EDGE_CURVE ( 'NONE', #3357, #4223, #5311, .T. ) ;
#11426=CARTESIAN_POINT ( 'NONE',  ( -15.27494751580540111, 73.62981360231496808, 9.945832149094092856 ) ) ;
#11427=DIRECTION ( 'NONE',  ( 1.000000000000000000, 6.033820786006286457E-17, -0.000000000000000000 ) ) ;
#11438=CARTESIAN_POINT ( 'NONE',  ( -30.33346888516166118, 47.99444905479163737, 0.0003276040068861179808 ) ) ;
#11440=LINE ( 'NONE', #3249, #1653 ) ;
#11448=CARTESIAN_POINT ( 'NONE',  ( 15.09270675947632689, 55.01153773592707097, -0.02355180096384254518 ) ) ;
#11456=CARTESIAN_POINT ( 'NONE',  ( -47.81092963715463640, 71.80394787507084686, -12.92116392654651058 ) ) ;
#11457=ORIENTED_EDGE ( 'NONE', *, *, #4529, .T. ) ;
#11458=CARTESIAN_POINT ( 'NONE',  ( 8.855705142202525693, 38.19481665208223120, 12.92224424505011271 ) ) ;
#11459=CARTESIAN_POINT ( 'NONE',  ( -4.539499248000766762, 53.16883361098971505, -13.98200185442132160 ) ) ;
#11462=CARTESIAN_POINT ( 'NONE',  ( -21.71149157619788994, 57.21358471493454090, 4.495333134771674288 ) ) ;
#11468=CARTESIAN_POINT ( 'NONE',  ( -52.91582296080724035, 62.01289876477373042, 0.6873062178531880173 ) ) ;
#11470=CARTESIAN_POINT ( 'NONE',  ( -56.05785376386896246, 64.93131079446247611, 18.59685268580366468 ) ) ;
#11472=CARTESIAN_POINT ( 'NONE',  ( 7.477680471578420196, 36.66673471410030061, 10.56605622896702990 ) ) ;
#11478=EDGE_LOOP ( 'NONE', ( #10012, #1090, #1523, #6262 ) ) ;
#11482=CARTESIAN_POINT ( 'NONE',  ( -29.26269115883859939, 34.87241548204915631, 6.108265559058850158 ) ) ;
#11500=CARTESIAN_POINT ( 'NONE',  ( -58.91624683120330275, 54.31316703610227847, 6.983828696265685920 ) ) ;
#11501=APPLICATION_CONTEXT ( 'automotive_design' ) ;
#11512=CARTESIAN_POINT ( 'NONE',  ( -15.99785213383137616, 55.00209440256361404, 0.002335802559052338814 ) ) ;
#11518=CARTESIAN_POINT ( 'NONE',  ( -52.27495405780593529, 76.01412898031726684, 2.059423305703688811 ) ) ;
#11520=CARTESIAN_POINT ( 'NONE',  ( -49.47762672124542149, 75.47109300164294154, -5.507530253420135580 ) ) ;
#11521=CARTESIAN_POINT ( 'NONE',  ( -9.121973149755229215, 63.34697924335122821, -11.25570253714172608 ) ) ;
#11525=CARTESIAN_POINT ( 'NONE',  ( 10.18903847268274276, 38.19250115101311849, 12.92455934260550521 ) ) ;
#11529=CARTESIAN_POINT ( 'NONE',  ( -45.62461256353399364, 57.99907488884235818, -6.340528469342151752 ) ) ;
#11531=CARTESIAN_POINT ( 'NONE',  ( -10.81092923698156838, 75.47407628921179423, -5.508885182882011122 ) ) ;
#11542=CARTESIAN_POINT ( 'NONE',  ( -30.40408068685511367, 34.08504365610654219, 2.058398070974400529 ) ) ;
#11545=VECTOR ( 'NONE', #5759, 1000.000000000000000 ) ;
#11546=CARTESIAN_POINT ( 'NONE',  ( 47.00000000000000000, 55.00000000000000000, 0.000000000000000000 ) ) ;
#11549=CARTESIAN_POINT ( 'NONE',  ( -36.85572911278101316, 38.22258139949027367, -12.89445763391127464 ) ) ;
#11557=CARTESIAN_POINT ( 'NONE',  ( -51.33319506590260062, 61.47761287630137161, 2.683395058215394702 ) ) ;
#11559=CARTESIAN_POINT ( 'NONE',  ( -13.54240173784083723, 59.84020960470326145, -1.295393626438009704 ) ) ;
#11576=CARTESIAN_POINT ( 'NONE',  ( -28.29255007849803860, 50.25485254516154043, 1.609630709827212236 ) ) ;
#11577=CARTESIAN_POINT ( 'NONE',  ( -57.50627882723209439, 66.73110044028416610, 17.54296274220338958 ) ) ;
#11579=CARTESIAN_POINT ( 'NONE',  ( -55.66294609945612137, 69.86598917288522159, 14.86507401989504373 ) ) ;
#11580=CARTESIAN_POINT ( 'NONE',  ( -6.496911930288724157, 57.74752198855276930, -13.79222801868778703 ) ) ;
#11589=CARTESIAN_POINT ( 'NONE',  ( -32.79192076745651008, 48.07125197820906237, 1.028503333593271174 ) ) ;
#11591=CARTESIAN_POINT ( 'NONE',  ( 1.608176249509176925, 38.70641480386327515, -13.38147628996001792 ) ) ;
#11597=SHAPE_REPRESENTATION ( 'Internal Tapered Feed Screw Auger', ( #4738 ), #7754 ) ;
#11602=CARTESIAN_POINT ( 'NONE',  ( -8.839809468419982608, 72.54364378520992318, -11.73195350307014273 ) ) ;
#11607=CARTESIAN_POINT ( 'NONE',  ( -68.37000832029607977, 50.50915739122872594, 2.223033420437384500 ) ) ;
#11609=PLANE ( 'NONE',  #2830 ) ;
#11610=CARTESIAN_POINT ( 'NONE',  ( -46.39182477221876866, 68.38321102182860045, -16.29532114285349920 ) ) ;
#11616=ORIENTED_EDGE ( 'NONE', *, *, #151, .F. ) ;
#11619=CARTESIAN_POINT ( 'NONE',  ( 24.53746899439483187, 69.02463592203230291, 1.835796648199006231 ) ) ;
#11630=CARTESIAN_POINT ( 'NONE',  ( 12.75940324669208792, 55.01967313903768542, -0.01734440949077138694 ) ) ;
#11633=CARTESIAN_POINT ( 'NONE',  ( -17.79452817730176406, 57.50745412809310864, 4.338269230264096166 ) ) ;
#11638=CARTESIAN_POINT ( 'NONE',  ( -32.63602705562564665, 33.99332947357206081, -1.031628927963774034 ) ) ;
#11639=CARTESIAN_POINT ( 'NONE',  ( -50.46043717566288933, 68.65163989201867878, -3.672846925086713288 ) ) ;
#11644=CARTESIAN_POINT ( 'NONE',  ( 4.595919313165082620, 34.88938507153989832, -6.102095433906166377 ) ) ;
#11652=CARTESIAN_POINT ( 'NONE',  ( 3.618939467528528020, 55.00553246306094479, 0.0003573287855505533355 ) ) ;
#11655=CARTESIAN_POINT ( 'NONE',  ( 23.52085514044975412, 76.02215512729939917, 2.750727249632518578 ) ) ;
#11656=CARTESIAN_POINT ( 'NONE',  ( -9.969360172258976860, 70.58303384883494402, -14.12411716821732277 ) ) ;
#11665=CARTESIAN_POINT ( 'NONE',  ( -34.85572910849313644, 38.22605186251247744, -12.89098713163435228 ) ) ;
#11669=ORIENTED_EDGE ( 'NONE', *, *, #7349, .F. ) ;
#11672=CARTESIAN_POINT ( 'NONE',  ( 18.34332550980965593, 58.97478973010875336, 3.050963776907112290 ) ) ;
#11679=CARTESIAN_POINT ( 'NONE',  ( 1.656070432594679565, 51.94480720268091289, -3.971655978929947484 ) ) ;
#11680=CARTESIAN_POINT ( 'NONE',  ( 12.87292705410422577, 47.94148912775095539, 12.25634023971492503 ) ) ;
#11689=EDGE_CURVE ( 'NONE', #760, #1948, #11123, .T. ) ;
#11697=CARTESIAN_POINT ( 'NONE',  ( -12.09272392674168017, 55.02619396104714866, 0.001659151704244336443 ) ) ;
#11705=CARTESIAN_POINT ( 'NONE',  ( -42.54809234475217039, 58.08538739954438057, -20.80116627830041054 ) ) ;
#11709=CARTESIAN_POINT ( 'NONE',  ( 18.81101721030213625, 65.56418867429738384, 18.32872549916029925 ) ) ;
#11710=ORIENTED_EDGE ( 'NONE', *, *, #9539, .F. ) ;
#11712=CARTESIAN_POINT ( 'NONE',  ( 15.64624132220377639, 54.34386165159118320, 4.967374051144239466 ) ) ;
#11713=CARTESIAN_POINT ( 'NONE',  ( -69.44401486253393330, 48.16327053899182431, 1.838581984797913460 ) ) ;
#11715=CARTESIAN_POINT ( 'NONE',  ( -62.51030605291772702, 43.28161195024001273, 17.55542603392786916 ) ) ;
#11716=CARTESIAN_POINT ( 'NONE',  ( -28.94161417925737823, 38.68453375511723635, 13.40299329694203578 ) ) ;
#11723=CARTESIAN_POINT ( 'NONE',  ( 36.99999999999999289, 59.99999999999998579, 0.000000000000000000 ) ) ;
#11724=PLANE ( 'NONE',  #8796 ) ;
#11726=CARTESIAN_POINT ( 'NONE',  ( -50.27495406422890767, 76.01781437481966464, 2.059423474151367728 ) ) ;
#11736=EDGE_LOOP ( 'NONE', ( #7362, #6784, #8100, #4015, #1078, #11710 ) ) ;
#11737=FACE_OUTER_BOUND ( 'NONE', #1187, .T. ) ;
#11740=CARTESIAN_POINT ( 'NONE',  ( -24.46043788332341151, 47.94142141767103737, 12.25631317379969509 ) ) ;
#11749=CARTESIAN_POINT ( 'NONE',  ( -40.20488286162279223, 55.00025610236561846, -0.004523070879801337381 ) ) ;
#11752=DIRECTION ( 'NONE',  ( 1.000000000000000000, 6.033820786006286457E-17, 0.000000000000000000 ) ) ;
#11755=EDGE_CURVE ( 'NONE', #3047, #2139, #4158, .T. ) ;
#11756=CARTESIAN_POINT ( 'NONE',  ( -30.59602397924764361, 34.87358162761611169, 6.107823804857911654 ) ) ;
#11758=MECHANICAL_DESIGN_GEOMETRIC_PRESENTATION_REPRESENTATION('',(#11169),#2199);
#11762=CARTESIAN_POINT ( 'NONE',  ( -18.45202553953894764, 65.80723110900194683, 18.02933743899848551 ) ) ;
#11765=CARTESIAN_POINT ( 'NONE',  ( -2.092693678294518467, 54.98959697584933792, -0.01274811450331606207 ) ) ;
#11766=VECTOR ( 'NONE', #2990, 1000.000000000000000 ) ;
#11768=CARTESIAN_POINT ( 'NONE',  ( -8.329477863459651132, 69.86497200091255877, -14.86570652194256148 ) ) ;
#11769=CARTESIAN_POINT ( 'NONE',  ( -15.85565286160008469, 75.43490621471428881, 5.492246195135631837 ) ) ;
#11771=DIRECTION ( 'NONE',  ( 0.000000000000000000, 1.000000000000000000, 0.000000000000000000 ) ) ;
#11781=CIRCLE ( 'NONE', #7970, 2.999999999999995559 ) ;
#11782=CARTESIAN_POINT ( 'NONE',  ( -53.98894970602387389, 59.83948248508205836, 1.298372112287061508 ) ) ;
#11787=EDGE_CURVE ( 'NONE', #1948, #4670, #10827, .T. ) ;
#11792=EDGE_CURVE ( 'NONE', #3881, #4551, #7326, .T. ) ;
#11798=CARTESIAN_POINT ( 'NONE',  ( -7.630320567153270339, 65.39170505435430414, -9.418633508564214551 ) ) ;
#11809=CARTESIAN_POINT ( 'NONE',  ( -59.75812396593624243, 55.00560539528500215, -0.01061549039029876899 ) ) ;
#11812=CARTESIAN_POINT ( 'NONE',  ( -18.95867291721290471, 56.61031706631060700, 4.744919608251485954 ) ) ;
#11816=CARTESIAN_POINT ( 'NONE',  ( -7.337209909475700620, 63.04728967918421745, -19.42673836724018699 ) ) ;
#11820=CARTESIAN_POINT ( 'NONE',  ( -30.40408068685511367, 34.08504365610654219, 2.058398070974400529 ) ) ;
#11824=CARTESIAN_POINT ( 'NONE',  ( -62.24957892231395817, 54.31321652181242854, 6.980810767642831927 ) ) ;
#11826=CARTESIAN_POINT ( 'NONE',  ( 22.81087673974644403, 75.43171151743705138, 5.491419164873361680 ) ) ;
#11827=CARTESIAN_POINT ( 'NONE',  ( -21.32947787934852357, 63.04568470447853912, 19.42265540296757464 ) ) ;
#11833=CARTESIAN_POINT ( 'NONE',  ( -47.43046783121353371, 54.99045398927809458, 0.007802215875459363355 ) ) ;
#11834=CARTESIAN_POINT ( 'NONE',  ( -55.71338727784861788, 57.06385637567746727, 4.557138327899026287 ) ) ;
#11836=DIRECTION ( 'NONE',  ( 0.000000000000000000, 1.000000000000000000, 0.000000000000000000 ) ) ;
#11840=DIRECTION ( 'NONE',  ( -1.000000000000000000, 0.000000000000000000, -0.000000000000000000 ) ) ;
#11842=CARTESIAN_POINT ( 'NONE',  ( 14.45936532742768321, 56.29682532305226772, 4.839835512798248196 ) ) ;
#11849=CARTESIAN_POINT ( 'NONE',  ( 0.8701179677062256257, 52.49160040349491396, -4.337762753772214985 ) ) ;
#11850=CARTESIAN_POINT ( 'NONE',  ( -3.830245506239644548, 57.74702083132989117, -13.79104772941276025 ) ) ;
#11852=CARTESIAN_POINT ( 'NONE',  ( 34.00000000000000000, 45.00000000000001421, 1.224646799147351679E-15 ) ) ;
#11889=COLOUR_RGB('Black',0.12,0.14,0.17);
#11890=FILL_AREA_STYLE_COLOUR('',#11889);
#11891=FILL_AREA_STYLE('',(#11890));
#11892=SURFACE_STYLE_FILL_AREA(#11891);
#11893=SURFACE_SIDE_STYLE('',(#11892));
#11894=SURFACE_STYLE_USAGE(.BOTH.,#11893);
#11895=PRESENTATION_STYLE_ASSIGNMENT((#11894));
ENDSEC;
END-ISO-10303-21;
